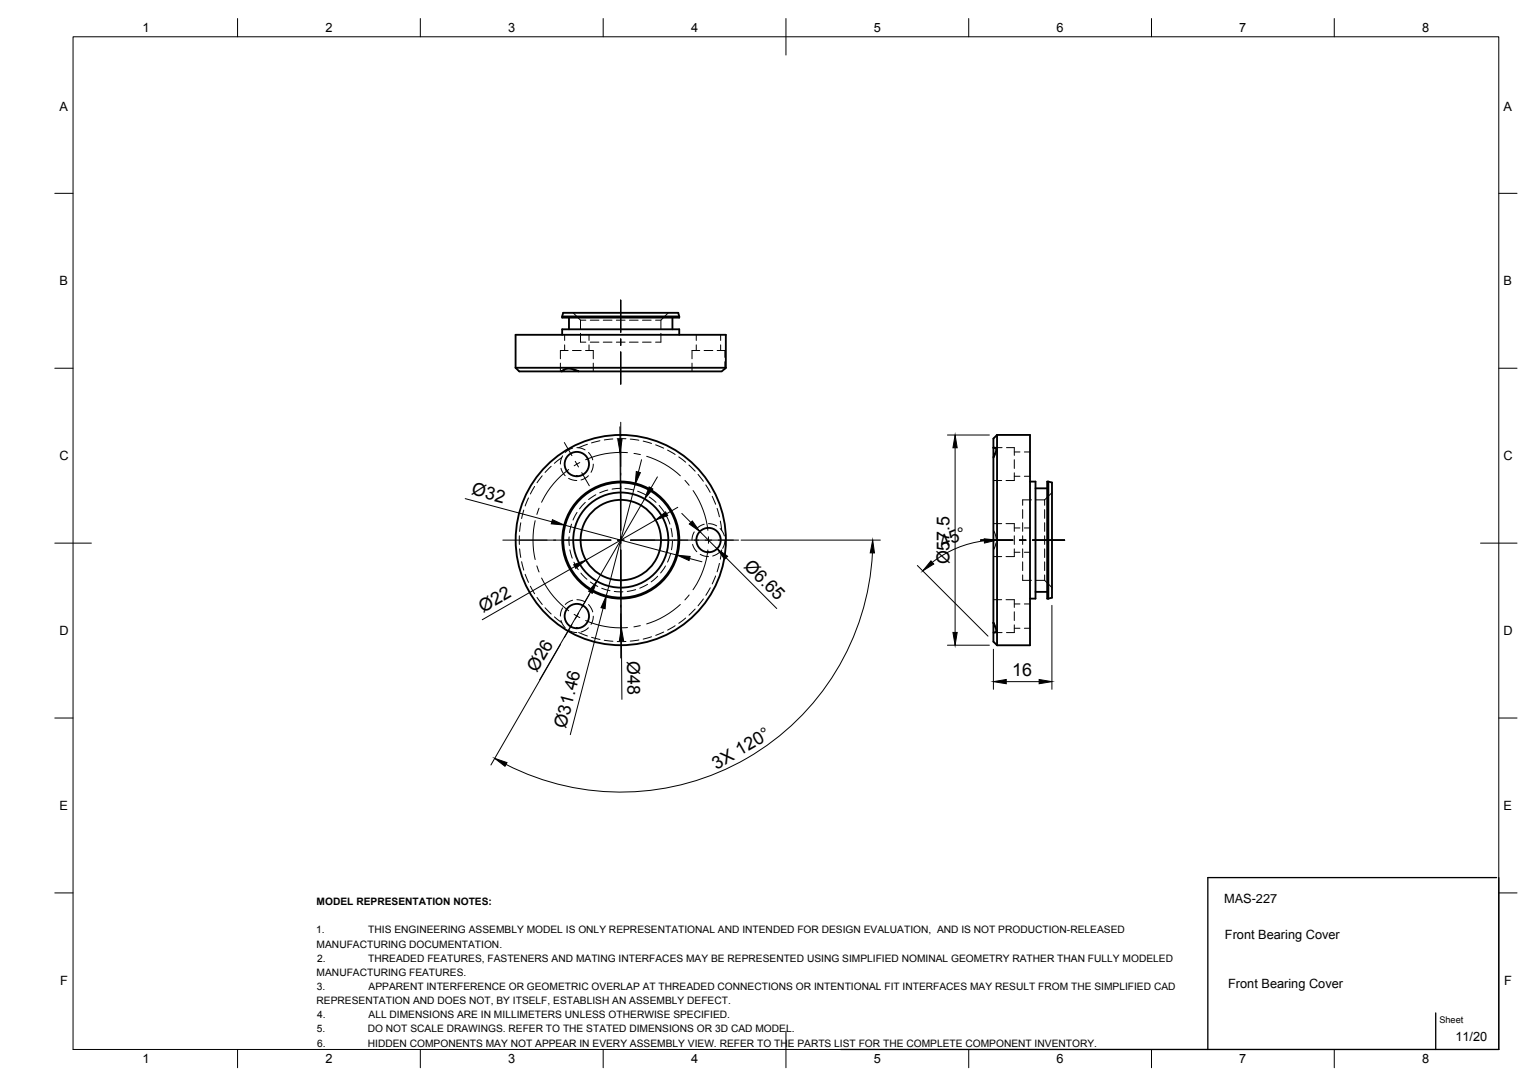
ISO-10303-21;
HEADER;
FILE_DESCRIPTION (('STEP AP214'),
    '1' );
FILE_NAME ( 'Front Bearing Cover.step', '2026-10-06T08:24:41', ( '' ), ( '' ), 'STEP AP214', 'Unspecified', '' );
FILE_SCHEMA (( 'AUTOMOTIVE_DESIGN' ));
ENDSEC;
DATA;
#2=LINE ( 'NONE', #16920, #12528 ) ;
#50=AXIS2_PLACEMENT_3D ( 'NONE', #26604, #25051, #22376 ) ;
#52=VECTOR ( 'NONE', #14977, 39.37007874015748143 ) ;
#127=DIRECTION ( 'NONE',  ( -1.000000000000000000, 0.000000000000000000, 0.000000000000000000 ) ) ;
#158=VERTEX_POINT ( 'NONE', #15724 ) ;
#172=CARTESIAN_POINT ( 'NONE',  ( -0.6029881478123397809, 1.118968434182175953, 0.03326447829408156476 ) ) ;
#190=CARTESIAN_POINT ( 'NONE',  ( -0.6299212598425196763, -0.4724409448818898127, -0.8182917201112815953 ) ) ;
#192=DIRECTION ( 'NONE',  ( -1.000000000000000000, 0.000000000000000000, 0.000000000000000000 ) ) ;
#253=DIRECTION ( 'NONE',  ( -1.000000000000000000, 0.000000000000000000, 0.000000000000000000 ) ) ;
#272=EDGE_CURVE ( 'NONE', #27250, #26868, #24521, .T. ) ;
#312=DIRECTION ( 'NONE',  ( 0.000000000000000000, 0.000000000000000000, 1.000000000000000000 ) ) ;
#392=ORIENTED_EDGE ( 'NONE', *, *, #12058, .F. ) ;
#416=EDGE_CURVE ( 'NONE', #7640, #15191, #10471, .T. ) ;
#433=DIRECTION ( 'NONE',  ( 1.000000000000000000, 0.000000000000000000, 0.000000000000000000 ) ) ;
#441=DIRECTION ( 'NONE',  ( 1.000000000000000000, 0.000000000000000000, 0.000000000000000000 ) ) ;
#479=CYLINDRICAL_SURFACE ( 'NONE', #571, 0.5570866141732283561 ) ;
#480=AXIS2_PLACEMENT_3D ( 'NONE', #1585, #2519, #13258 ) ;
#513=ORIENTED_EDGE ( 'NONE', *, *, #2642, .T. ) ;
#528=EDGE_LOOP ( 'NONE', ( #9986, #24877, #1531, #26427 ) ) ;
#562=FACE_OUTER_BOUND ( 'NONE', #19020, .T. ) ;
#571=AXIS2_PLACEMENT_3D ( 'NONE', #26308, #7804, #10047 ) ;
#585=EDGE_CURVE ( 'NONE', #20760, #20801, #19125, .T. ) ;
#624=CARTESIAN_POINT ( 'NONE',  ( -0.6020308615105518513, -0.5839868939189144514, 0.9562171551411200454 ) ) ;
#670=AXIS2_PLACEMENT_3D ( 'NONE', #15079, #14812, #19294 ) ;
#698=CIRCLE ( 'NONE', #4312, 0.5570866141732283561 ) ;
#725=ORIENTED_EDGE ( 'NONE', *, *, #8155, .T. ) ;
#767=EDGE_CURVE ( 'NONE', #19729, #5602, #7540, .T. ) ;
#774=LINE ( 'NONE', #17967, #26208 ) ;
#782=CYLINDRICAL_SURFACE ( 'NONE', #20278, 0.4330708661417322913 ) ;
#838=EDGE_CURVE ( 'NONE', #4142, #1699, #4370, .T. ) ;
#875=EDGE_CURVE ( 'NONE', #4894, #7494, #21145, .T. ) ;
#905=CARTESIAN_POINT ( 'NONE',  ( -0.1771653543307086520, 0.5935039370078740717, 0.000000000000000000 ) ) ;
#906=ORIENTED_EDGE ( 'NONE', *, *, #6294, .T. ) ;
#913=FACE_OUTER_BOUND ( 'NONE', #10036, .T. ) ;
#918=VECTOR ( 'NONE', #23051, 39.37007874015748143 ) ;
#928=EDGE_CURVE ( 'NONE', #158, #23473, #6082, .T. ) ;
#936=AXIS2_PLACEMENT_3D ( 'NONE', #3031, #24513, #15779 ) ;
#939=CARTESIAN_POINT ( 'NONE',  ( -0.6299212598425196763, 1.087444635826771533, -0.1051828227901515783 ) ) ;
#940=FACE_OUTER_BOUND ( 'NONE', #528, .T. ) ;
#951=VECTOR ( 'NONE', #3285, 39.37007874015748143 ) ;
#1039=DIRECTION ( 'NONE',  ( 0.000000000000000000, 0.000000000000000000, 1.000000000000000000 ) ) ;
#1046=DIRECTION ( 'NONE',  ( 0.000000000000000000, 0.000000000000000000, 1.000000000000000000 ) ) ;
#1048=AXIS2_PLACEMENT_3D ( 'NONE', #23857, #19612, #2759 ) ;
#1080=CONICAL_SURFACE ( 'NONE', #17752, 0.6246466694403326469, 0.2617993874999998694 ) ;
#1092=ORIENTED_EDGE ( 'NONE', *, *, #1886, .F. ) ;
#1098=( NAMED_UNIT ( * ) PLANE_ANGLE_UNIT ( ) SI_UNIT ( $, .RADIAN. ) ) ;
#1120=FACE_OUTER_BOUND ( 'NONE', #1478, .T. ) ;
#1124=AXIS2_PLACEMENT_3D ( 'NONE', #13348, #15489, #11366 ) ;
#1198=DIRECTION ( 'NONE',  ( -1.000000000000000000, 0.000000000000000000, 0.000000000000000000 ) ) ;
#1239=CARTESIAN_POINT ( 'NONE',  ( -0.1141732283464566844, 0.000000000000000000, 0.000000000000000000 ) ) ;
#1283=VECTOR ( 'NONE', #10032, 39.37007874015748143 ) ;
#1301=AXIS2_PLACEMENT_3D ( 'NONE', #19572, #253, #4583 ) ;
#1342=VERTEX_POINT ( 'NONE', #2206 ) ;
#1346=ORIENTED_EDGE ( 'NONE', *, *, #7162, .F. ) ;
#1382=DIRECTION ( 'NONE',  ( -1.000000000000000000, 0.000000000000000000, 0.000000000000000000 ) ) ;
#1478=EDGE_LOOP ( 'NONE', ( #8404, #19161 ) ) ;
#1485=ORIENTED_EDGE ( 'NONE', *, *, #4157, .T. ) ;
#1531=ORIENTED_EDGE ( 'NONE', *, *, #24469, .T. ) ;
#1570=DIRECTION ( 'NONE',  ( 1.000000000000000000, 0.000000000000000000, 0.000000000000000000 ) ) ;
#1571=CIRCLE ( 'NONE', #24136, 0.1771653543307086798 ) ;
#1585=CARTESIAN_POINT ( 'NONE',  ( -0.1771653543307086520, 0.000000000000000000, 0.000000000000000000 ) ) ;
#1644=FACE_OUTER_BOUND ( 'NONE', #10088, .T. ) ;
#1657=PRODUCT_CONTEXT ( 'NONE', #12864, 'mechanical' ) ;
#1699=VERTEX_POINT ( 'NONE', #13055 ) ;
#1701=DIRECTION ( 'NONE',  ( -0.9659258263664939337, -0.2588190448135644917, 0.000000000000000000 ) ) ;
#1711=ORIENTED_EDGE ( 'NONE', *, *, #11780, .F. ) ;
#1740=CARTESIAN_POINT ( 'NONE',  ( -0.6071192803969113205, -0.6030946203081917201, -0.9382345488190140248 ) ) ;
#1753=CIRCLE ( 'NONE', #25681, 0.5118110236220472231 ) ;
#1777=CARTESIAN_POINT ( 'NONE',  ( 2.632951206231566310, -0.4724409448818898127, 0.6874452634183660926 ) ) ;
#1827=FACE_OUTER_BOUND ( 'NONE', #23500, .T. ) ;
#1877=DIRECTION ( 'NONE',  ( 0.000000000000000000, 0.000000000000000000, 1.000000000000000000 ) ) ;
#1881=CARTESIAN_POINT ( 'NONE',  ( -0.6138531223217379429, -0.4891464190266830436, -0.9948699164928014316 ) ) ;
#1886=EDGE_CURVE ( 'NONE', #7494, #4592, #5665, .T. ) ;
#1902=CARTESIAN_POINT ( 'NONE',  ( -0.6086685665488132946, -0.5056997808540499850, 0.9923580223642571863 ) ) ;
#1968=CARTESIAN_POINT ( 'NONE',  ( -0.6299212598425196763, -0.4724409448818898127, 0.6411263657805708061 ) ) ;
#1969=DIRECTION ( 'NONE',  ( 0.000000000000000000, 1.000000000000000000, 0.000000000000000000 ) ) ;
#1976=ORIENTED_EDGE ( 'NONE', *, *, #15552, .T. ) ;
#1989=CARTESIAN_POINT ( 'NONE',  ( -0.6299212598425196763, -1.092519685074702762, 0.000000000000000000 ) ) ;
#1992=CYLINDRICAL_SURFACE ( 'NONE', #10340, 0.1771653543307086798 ) ;
#2006=CARTESIAN_POINT ( 'NONE',  ( -0.2066929133858267931, 0.6299212598425196763, 0.000000000000000000 ) ) ;
#2020=AXIS2_PLACEMENT_3D ( 'NONE', #5757, #7869, #12099 ) ;
#2023=CARTESIAN_POINT ( 'NONE',  ( -0.6205631318075456315, -0.4724394499398413827, -0.9954595798869798617 ) ) ;
#2029=DIMENSIONAL_EXPONENTS ( 1.000000000000000000, 0.000000000000000000, 0.000000000000000000, 0.000000000000000000, 0.000000000000000000, 0.000000000000000000, 0.000000000000000000 ) ;
#2047=ORIENTED_EDGE ( 'NONE', *, *, #11733, .T. ) ;
#2096=ORIENTED_EDGE ( 'NONE', *, *, #13801, .T. ) ;
#2101=CARTESIAN_POINT ( 'NONE',  ( -0.3149606299212598381, 0.000000000000000000, 0.000000000000000000 ) ) ;
#2149=EDGE_CURVE ( 'NONE', #23473, #158, #698, .T. ) ;
#2157=ORIENTED_EDGE ( 'NONE', *, *, #18019, .T. ) ;
#2175=EDGE_CURVE ( 'NONE', #3772, #3172, #5916, .T. ) ;
#2206=CARTESIAN_POINT ( 'NONE',  ( -0.6299212598425196763, -0.6348133144914134274, -0.8891632684400255782 ) ) ;
#2228=ORIENTED_EDGE ( 'NONE', *, *, #17985, .F. ) ;
#2241=CARTESIAN_POINT ( 'NONE',  ( -0.6003937007829848183, 1.122047244090071727, 1.315345636034250449E-15 ) ) ;
#2293=EDGE_CURVE ( 'NONE', #20801, #20760, #12897, .T. ) ;
#2306=LINE ( 'NONE', #17693, #23561 ) ;
#2317=VERTEX_POINT ( 'NONE', #19276 ) ;
#2319=CYLINDRICAL_SURFACE ( 'NONE', #1301, 0.1308464566929133932 ) ;
#2341=CYLINDRICAL_SURFACE ( 'NONE', #16764, 0.1308464566929133932 ) ;
#2355=FACE_OUTER_BOUND ( 'NONE', #2723, .T. ) ;
#2398=CARTESIAN_POINT ( 'NONE',  ( -0.5177165354330708347, -0.4724409448818898127, 0.6411263657805708061 ) ) ;
#2414=LINE ( 'NONE', #2006, #23718 ) ;
#2449=EDGE_CURVE ( 'NONE', #14962, #17328, #26863, .T. ) ;
#2473=ORIENTED_EDGE ( 'NONE', *, *, #20578, .F. ) ;
#2475=VECTOR ( 'NONE', #16821, 39.37007874015748143 ) ;
#2519=DIRECTION ( 'NONE',  ( 1.000000000000000000, 0.000000000000000000, 0.000000000000000000 ) ) ;
#2526=DIRECTION ( 'NONE',  ( 1.000000000000000000, 0.000000000000000000, 0.000000000000000000 ) ) ;
#2535=CARTESIAN_POINT ( 'NONE',  ( -0.6299212598425196763, -0.4526313213353582721, -0.9943460912301771426 ) ) ;
#2600=DIRECTION ( 'NONE',  ( 0.000000000000000000, 0.000000000000000000, 1.000000000000000000 ) ) ;
#2609=DIRECTION ( 'NONE',  ( 1.000000000000000000, 0.000000000000000000, 0.000000000000000000 ) ) ;
#2618=ORIENTED_EDGE ( 'NONE', *, *, #8797, .T. ) ;
#2630=CARTESIAN_POINT ( 'NONE',  ( -0.2362204724409449064, 0.9448818897637796255, 0.1308464566929133654 ) ) ;
#2635=ORIENTED_EDGE ( 'NONE', *, *, #16037, .F. ) ;
#2642=EDGE_CURVE ( 'NONE', #5602, #25182, #2, .T. ) ;
#2720=EDGE_CURVE ( 'NONE', #5602, #19729, #7100, .T. ) ;
#2723=EDGE_LOOP ( 'NONE', ( #26638, #22078, #16466, #23009 ) ) ;
#2759=DIRECTION ( 'NONE',  ( 0.000000000000000000, 0.000000000000000000, -1.000000000000000000 ) ) ;
#2778=EDGE_CURVE ( 'NONE', #26868, #27250, #21542, .T. ) ;
#2786=CARTESIAN_POINT ( 'NONE',  ( -0.03937007874015747977, 0.000000000000000000, 0.000000000000000000 ) ) ;
#2850=PLANE ( 'NONE',  #16081 ) ;
#2955=CYLINDRICAL_SURFACE ( 'NONE', #4382, 0.6299212598425196763 ) ;
#2956=ADVANCED_FACE ( 'NONE', ( #9507, #11506 ), #18107, .T. ) ;
#3017=ORIENTED_EDGE ( 'NONE', *, *, #6004, .T. ) ;
#3031=CARTESIAN_POINT ( 'NONE',  ( -0.05118110236220472370, 0.000000000000000000, 0.000000000000000000 ) ) ;
#3041=DIRECTION ( 'NONE',  ( 0.000000000000000000, 1.000000000000000000, 0.000000000000000000 ) ) ;
#3045=SURFACE_SIDE_STYLE ('',( #5177 ) ) ;
#3076=MANIFOLD_SOLID_BREP ( 'Front Bearing Cover', #11437 ) ;
#3092=DIRECTION ( 'NONE',  ( 0.000000000000000000, 1.000000000000000000, 0.000000000000000000 ) ) ;
#3147=FACE_OUTER_BOUND ( 'NONE', #4581, .T. ) ;
#3157=PRODUCT_DEFINITION_CONTEXT ( 'detailed design', #6031, 'design' ) ;
#3162=DIRECTION ( 'NONE',  ( 0.7071067818211385081, 0.7071067805519564153, -8.659560554583433905E-17 ) ) ;
#3165=AXIS2_PLACEMENT_3D ( 'NONE', #26491, #11954, #22410 ) ;
#3169=DIRECTION ( 'NONE',  ( 0.000000000000000000, 0.000000000000000000, 1.000000000000000000 ) ) ;
#3172=VERTEX_POINT ( 'NONE', #20257 ) ;
#3176=ORIENTED_EDGE ( 'NONE', *, *, #19126, .T. ) ;
#3186=CYLINDRICAL_SURFACE ( 'NONE', #8980, 0.5570866141732283561 ) ;
#3280=CIRCLE ( 'NONE', #22700, 0.1771653543307086798 ) ;
#3285=DIRECTION ( 'NONE',  ( -1.000000000000000000, 0.000000000000000000, 0.000000000000000000 ) ) ;
#3289=ORIENTED_EDGE ( 'NONE', *, *, #7803, .T. ) ;
#3334=CARTESIAN_POINT ( 'NONE',  ( 1.857656692913385893E-16, 0.6193720790381457286, 7.649715443242610847E-17 ) ) ;
#3339=AXIS2_PLACEMENT_3D ( 'NONE', #27556, #6091, #1969 ) ;
#3421=PLANE ( 'NONE',  #6401 ) ;
#3458=CARTESIAN_POINT ( 'NONE',  ( -0.07874015748031495954, 0.000000000000000000, 0.000000000000000000 ) ) ;
#3556=CARTESIAN_POINT ( 'NONE',  ( -0.02559055118110236185, -0.6299212598425196763, 7.714310545810098438E-17 ) ) ;
#3561=DIRECTION ( 'NONE',  ( -1.000000000000000000, 0.000000000000000000, 0.000000000000000000 ) ) ;
#3634=CARTESIAN_POINT ( 'NONE',  ( -0.5905511811023621549, 0.000000000000000000, 0.000000000000000000 ) ) ;
#3665=DIRECTION ( 'NONE',  ( 0.000000000000000000, 0.000000000000000000, 1.000000000000000000 ) ) ;
#3691=PRODUCT ( 'Front Bearing Cover', 'Front Bearing Cover', '', ( #1657 ) ) ;
#3700=VECTOR ( 'NONE', #23424, 39.37007874015748143 ) ;
#3772=VERTEX_POINT ( 'NONE', #20861 ) ;
#3862=CARTESIAN_POINT ( 'NONE',  ( -0.6086690512655491547, -0.5056979702033415069, -0.9923584033843172447 ) ) ;
#3879=EDGE_CURVE ( 'NONE', #13155, #23967, #1753, .T. ) ;
#3884=ORIENTED_EDGE ( 'NONE', *, *, #5984, .T. ) ;
#3919=CARTESIAN_POINT ( 'NONE',  ( -0.2362204724409449064, -1.131889763779527547, 1.386165176200252194E-16 ) ) ;
#3977=CARTESIAN_POINT ( 'NONE',  ( -0.4055118110236220486, -0.4724409448818898127, -0.8182917201112815953 ) ) ;
#4009=CARTESIAN_POINT ( 'NONE',  ( -0.6050289243185338339, -0.5969388012301621860, -0.9446411342989878834 ) ) ;
#4010=AXIS2_PLACEMENT_3D ( 'NONE', #17654, #27861, #13413 ) ;
#4032=EDGE_LOOP ( 'NONE', ( #13615, #17061 ) ) ;
#4033=ORIENTED_EDGE ( 'NONE', *, *, #2149, .F. ) ;
#4039=AXIS2_PLACEMENT_3D ( 'NONE', #2786, #15416, #312 ) ;
#4052=DIRECTION ( 'NONE',  ( 0.000000000000000000, -1.000000000000000000, 0.000000000000000000 ) ) ;
#4058=ORIENTED_EDGE ( 'NONE', *, *, #13801, .F. ) ;
#4088=CARTESIAN_POINT ( 'NONE',  ( -0.05118110236220472370, 0.5570866141732283561, 0.000000000000000000 ) ) ;
#4100=AXIS2_PLACEMENT_3D ( 'NONE', #11265, #13943, #7163 ) ;
#4142=VERTEX_POINT ( 'NONE', #15662 ) ;
#4157=EDGE_CURVE ( 'NONE', #15892, #26494, #5820, .T. ) ;
#4227=DIRECTION ( 'NONE',  ( 1.000000000000000000, 0.000000000000000000, 0.000000000000000000 ) ) ;
#4284=ORIENTED_EDGE ( 'NONE', *, *, #8725, .T. ) ;
#4304=DIRECTION ( 'NONE',  ( -1.000000000000000000, 0.000000000000000000, 0.000000000000000000 ) ) ;
#4311=EDGE_CURVE ( 'NONE', #19874, #10834, #13049, .T. ) ;
#4312=AXIS2_PLACEMENT_3D ( 'NONE', #13964, #10269, #16225 ) ;
#4370=LINE ( 'NONE', #13117, #25467 ) ;
#4382=AXIS2_PLACEMENT_3D ( 'NONE', #11586, #24576, #3092 ) ;
#4397=ADVANCED_FACE ( 'NONE', ( #21355 ), #1992, .F. ) ;
#4430=CARTESIAN_POINT ( 'NONE',  ( -0.6299212598425196763, 1.087444635826771533, -0.1051828227901515783 ) ) ;
#4453=ORIENTED_EDGE ( 'NONE', *, *, #16423, .F. ) ;
#4499=CARTESIAN_POINT ( 'NONE',  ( -0.6299212598425196763, 0.000000000000000000, 0.000000000000000000 ) ) ;
#4523=CARTESIAN_POINT ( 'NONE',  ( -0.6299212598425196763, 0.000000000000000000, 0.000000000000000000 ) ) ;
#4564=DIRECTION ( 'NONE',  ( -1.000000000000000000, 0.000000000000000000, 0.000000000000000000 ) ) ;
#4581=EDGE_LOOP ( 'NONE', ( #20664, #22877 ) ) ;
#4583=DIRECTION ( 'NONE',  ( 0.000000000000000000, 0.000000000000000000, -1.000000000000000000 ) ) ;
#4592=VERTEX_POINT ( 'NONE', #13879 ) ;
#4629=AXIS2_PLACEMENT_3D ( 'NONE', #11749, #5251, #25164 ) ;
#4647=ORIENTED_EDGE ( 'NONE', *, *, #24298, .T. ) ;
#4661=DIRECTION ( 'NONE',  ( -1.000000000000000000, 0.000000000000000000, 0.000000000000000000 ) ) ;
#4671=CIRCLE ( 'NONE', #19590, 1.131889763779527547 ) ;
#4677=CYLINDRICAL_SURFACE ( 'NONE', #19084, 0.1308464566929133932 ) ;
#4704=ORIENTED_EDGE ( 'NONE', *, *, #272, .F. ) ;
#4711=FACE_OUTER_BOUND ( 'NONE', #27003, .T. ) ;
#4795=VERTEX_POINT ( 'NONE', #8631 ) ;
#4815=ORIENTED_EDGE ( 'NONE', *, *, #20578, .T. ) ;
#4843=CARTESIAN_POINT ( 'NONE',  ( -0.6002206662457667541, -0.5625442442678819654, 0.9710808210061889767 ) ) ;
#4867=MECHANICAL_DESIGN_GEOMETRIC_PRESENTATION_REPRESENTATION('',(#9349),#13888);
#4879=EDGE_LOOP ( 'NONE', ( #13228, #15107, #14974, #9118 ) ) ;
#4894=VERTEX_POINT ( 'NONE', #6696 ) ;
#4897=CIRCLE ( 'NONE', #4010, 0.1308464566929133932 ) ;
#4929=AXIS2_PLACEMENT_3D ( 'NONE', #19766, #433, #15543 ) ;
#4945=DIRECTION ( 'NONE',  ( -1.000000000000000000, 0.000000000000000000, 0.000000000000000000 ) ) ;
#5070=CARTESIAN_POINT ( 'NONE',  ( -0.2362204724409449064, 1.131889763779527547, 0.000000000000000000 ) ) ;
#5085=AXIS2_PLACEMENT_3D ( 'NONE', #24163, #22043, #26013 ) ;
#5128=DIRECTION ( 'NONE',  ( 0.000000000000000000, 0.000000000000000000, -1.000000000000000000 ) ) ;
#5156=CARTESIAN_POINT ( 'NONE',  ( -0.6209926255554318875, 1.097802432539390916, -0.08994119036278866441 ) ) ;
#5177=SURFACE_STYLE_FILL_AREA ( #25489 ) ;
#5196=DIRECTION ( 'NONE',  ( 0.000000000000000000, -1.000000000000000000, 0.000000000000000000 ) ) ;
#5229=CARTESIAN_POINT ( 'NONE',  ( 0.000000000000000000, 0.000000000000000000, 0.000000000000000000 ) ) ;
#5246=ORIENTED_EDGE ( 'NONE', *, *, #416, .F. ) ;
#5251=DIRECTION ( 'NONE',  ( -1.000000000000000000, 0.000000000000000000, 0.000000000000000000 ) ) ;
#5303=CARTESIAN_POINT ( 'NONE',  ( -0.6130487771524342211, 1.107101695598143642, -0.07148403028289961048 ) ) ;
#5379=DIRECTION ( 'NONE',  ( -1.000000000000000000, 0.000000000000000000, 0.000000000000000000 ) ) ;
#5451=ORIENTED_EDGE ( 'NONE', *, *, #16037, .T. ) ;
#5452=EDGE_LOOP ( 'NONE', ( #15442, #19741 ) ) ;
#5489=VERTEX_POINT ( 'NONE', #18159 ) ;
#5490=CARTESIAN_POINT ( 'NONE',  ( 1.877524803149606209E-16, 5.303588500244442984E-17, -0.4330708661417322913 ) ) ;
#5519=ORIENTED_EDGE ( 'NONE', *, *, #12634, .F. ) ;
#5566=CARTESIAN_POINT ( 'NONE',  ( -0.02559055118110236185, 0.000000000000000000, 0.000000000000000000 ) ) ;
#5575=CARTESIAN_POINT ( 'NONE',  ( -0.07874015748031495954, 0.000000000000000000, 0.4330708661417322913 ) ) ;
#5596=DIRECTION ( 'NONE',  ( -1.000000000000000000, 0.000000000000000000, 0.000000000000000000 ) ) ;
#5602=VERTEX_POINT ( 'NONE', #3334 ) ;
#5617=EDGE_CURVE ( 'NONE', #9929, #1699, #22039, .T. ) ;
#5633=FACE_BOUND ( 'NONE', #5452, .T. ) ;
#5639=VECTOR ( 'NONE', #127, 39.37007874015748143 ) ;
#5665=CIRCLE ( 'NONE', #24152, 0.1771653543307086520 ) ;
#5671=ORIENTED_EDGE ( 'NONE', *, *, #9315, .F. ) ;
#5727=ORIENTED_EDGE ( 'NONE', *, *, #19126, .F. ) ;
#5757=CARTESIAN_POINT ( 'NONE',  ( -0.6299212598425196763, 0.9448818897637796255, -9.561468503937007847E-18 ) ) ;
#5784=VERTEX_POINT ( 'NONE', #18914 ) ;
#5798=DIRECTION ( 'NONE',  ( 0.7071067818211390632, -8.659560554583428975E-17, -0.7071067805519560823 ) ) ;
#5817=AXIS2_PLACEMENT_3D ( 'NONE', #2101, #10713, #12965 ) ;
#5820=CIRCLE ( 'NONE', #13027, 0.6299212598425196763 ) ;
#5827=VERTEX_POINT ( 'NONE', #1968 ) ;
#5856=LINE ( 'NONE', #7831, #22622 ) ;
#5895=FACE_BOUND ( 'NONE', #4032, .T. ) ;
#5916=LINE ( 'NONE', #5490, #20087 ) ;
#5984=EDGE_CURVE ( 'NONE', #10834, #19874, #22524, .T. ) ;
#6004=EDGE_CURVE ( 'NONE', #27250, #20760, #8800, .T. ) ;
#6031=APPLICATION_CONTEXT ( 'automotive_design' ) ;
#6082=CIRCLE ( 'NONE', #3339, 0.5570866141732283561 ) ;
#6091=DIRECTION ( 'NONE',  ( 1.000000000000000000, 0.000000000000000000, 0.000000000000000000 ) ) ;
#6114=EDGE_LOOP ( 'NONE', ( #20873, #27817 ) ) ;
#6130=CIRCLE ( 'NONE', #15600, 0.6299212598425196763 ) ;
#6134=CIRCLE ( 'NONE', #20997, 0.6299212598425196763 ) ;
#6141=CARTESIAN_POINT ( 'NONE',  ( -0.6010693932361863556, -0.5770964849832589394, -0.9615141454542482924 ) ) ;
#6152=ORIENTED_EDGE ( 'NONE', *, *, #19042, .F. ) ;
#6181=B_SPLINE_CURVE_WITH_KNOTS ( 'NONE', 3,
 ( #10656, #23399, #12643, #21270, #1902, #19277, #10515, #19134, #27768, #4843, #19830, #624, #17697, #13186, #17432, #26050, #15347 ),
 .UNSPECIFIED., .F., .F.,
 ( 4, 2, 2, 1, 2, 2, 2, 2, 4 ),
 ( 0.08984410251848014284, 0.2036135897036702169, 0.2604983332962649833, 0.3173830768888596943, 0.4311525640740497822, 0.5449220512592398702, 0.6586915384444299582, 0.7724610256296200461, 1.000000000000000000 ),
 .UNSPECIFIED. ) ;
#6196=FACE_OUTER_BOUND ( 'NONE', #21586, .T. ) ;
#6214=EDGE_CURVE ( 'NONE', #25955, #13695, #25285, .T. ) ;
#6222=CARTESIAN_POINT ( 'NONE',  ( -0.6042043723480865491, 1.117528104686773327, 0.04027680511324581436 ) ) ;
#6269=DIRECTION ( 'NONE',  ( 1.000000000000000000, 0.000000000000000000, 0.000000000000000000 ) ) ;
#6281=ADVANCED_FACE ( 'NONE', ( #12240 ), #3186, .T. ) ;
#6294=EDGE_CURVE ( 'NONE', #5784, #2317, #11684, .T. ) ;
#6306=DIRECTION ( 'NONE',  ( 0.000000000000000000, 0.000000000000000000, 1.000000000000000000 ) ) ;
#6348=CARTESIAN_POINT ( 'NONE',  ( 2.632951206231566310, 0.9448818897637796255, -0.1308464566929134210 ) ) ;
#6370=ORIENTED_EDGE ( 'NONE', *, *, #25909, .F. ) ;
#6401=AXIS2_PLACEMENT_3D ( 'NONE', #11778, #20397, #18398 ) ;
#6426=DIRECTION ( 'NONE',  ( -1.000000000000000000, 0.000000000000000000, 0.000000000000000000 ) ) ;
#6443=DIRECTION ( 'NONE',  ( 0.000000000000000000, 0.000000000000000000, -1.000000000000000000 ) ) ;
#6452=DIRECTION ( 'NONE',  ( -0.9659258263664939337, 0.2588190448135644917, 3.169619147893071122E-17 ) ) ;
#6487=ADVANCED_FACE ( 'NONE', ( #7002 ), #8554, .T. ) ;
#6551=DIRECTION ( 'NONE',  ( -1.000000000000000000, 0.000000000000000000, 0.000000000000000000 ) ) ;
#6575=ADVANCED_FACE ( 'NONE', ( #11096 ), #782, .F. ) ;
#6696=CARTESIAN_POINT ( 'NONE',  ( -0.6003937007829848183, 1.122047244090071727, 1.315345636034250449E-15 ) ) ;
#6708=DIRECTION ( 'NONE',  ( 1.000000000000000000, 0.000000000000000000, 0.000000000000000000 ) ) ;
#6710=CARTESIAN_POINT ( 'NONE',  ( -0.4055118110236220486, -0.4724409448818898127, 0.8182917201112794858 ) ) ;
#6771=ORIENTED_EDGE ( 'NONE', *, *, #12058, .T. ) ;
#6778=DIRECTION ( 'NONE',  ( 0.000000000000000000, 1.000000000000000000, 0.000000000000000000 ) ) ;
#6781=FACE_OUTER_BOUND ( 'NONE', #9892, .T. ) ;
#6790=ORIENTED_EDGE ( 'NONE', *, *, #21213, .T. ) ;
#6805=EDGE_CURVE ( 'NONE', #12305, #4795, #15787, .T. ) ;
#6813=ORIENTED_EDGE ( 'NONE', *, *, #4157, .F. ) ;
#6821=ORIENTED_EDGE ( 'NONE', *, *, #10361, .T. ) ;
#6866=ORIENTED_EDGE ( 'NONE', *, *, #9739, .T. ) ;
#6895=LINE ( 'NONE', #15525, #20299 ) ;
#6932=CIRCLE ( 'NONE', #7357, 0.5570866141732283561 ) ;
#6950=VECTOR ( 'NONE', #5798, 39.37007874015748143 ) ;
#6998=DIRECTION ( 'NONE',  ( 0.000000000000000000, 0.000000000000000000, -1.000000000000000000 ) ) ;
#7002=FACE_OUTER_BOUND ( 'NONE', #15517, .T. ) ;
#7024=CARTESIAN_POINT ( 'NONE',  ( -0.2066929133858267931, 0.000000000000000000, 0.000000000000000000 ) ) ;
#7061=ORIENTED_EDGE ( 'NONE', *, *, #8900, .T. ) ;
#7074=CARTESIAN_POINT ( 'NONE',  ( -0.5905511811023621549, -1.131889763779527547, 1.386165176200252194E-16 ) ) ;
#7082=EDGE_CURVE ( 'NONE', #4795, #4592, #6895, .T. ) ;
#7100=CIRCLE ( 'NONE', #14817, 0.6193720790381457286 ) ;
#7102=DIRECTION ( 'NONE',  ( -1.000000000000000000, 0.000000000000000000, 0.000000000000000000 ) ) ;
#7143=CARTESIAN_POINT ( 'NONE',  ( -0.6205616028481958368, -0.4724399524669597450, 0.9954595399567032210 ) ) ;
#7152=AXIS2_PLACEMENT_3D ( 'NONE', #15250, #21737, #17080 ) ;
#7162=EDGE_CURVE ( 'NONE', #26868, #20801, #19748, .T. ) ;
#7163=DIRECTION ( 'NONE',  ( 0.000000000000000000, 0.000000000000000000, 1.000000000000000000 ) ) ;
#7234=ADVANCED_FACE ( 'NONE', ( #13652 ), #26641, .F. ) ;
#7238=CARTESIAN_POINT ( 'NONE',  ( -0.4055118110236220486, -0.4724409448818898127, -0.6411263657805729155 ) ) ;
#7241=DIRECTION ( 'NONE',  ( 0.000000000000000000, 0.000000000000000000, 1.000000000000000000 ) ) ;
#7288=FACE_OUTER_BOUND ( 'NONE', #19185, .T. ) ;
#7315=ORIENTED_EDGE ( 'NONE', *, *, #2449, .F. ) ;
#7339=ADVANCED_FACE ( 'NONE', ( #23454 ), #23862, .T. ) ;
#7344=UNCERTAINTY_MEASURE_WITH_UNIT (LENGTH_MEASURE( 1.000000000000000082E-05 ), #9669, 'distance_accuracy_value', 'NONE') ;
#7357=AXIS2_PLACEMENT_3D ( 'NONE', #26685, #22598, #20624 ) ;
#7370=AXIS2_PLACEMENT_3D ( 'NONE', #26123, #20035, #6778 ) ;
#7395=DIRECTION ( 'NONE',  ( 0.000000000000000000, 1.000000000000000000, 0.000000000000000000 ) ) ;
#7418=CARTESIAN_POINT ( 'NONE',  ( -0.6094642026423211512, 1.111319899719084070, -0.06074667524627151011 ) ) ;
#7467=EDGE_LOOP ( 'NONE', ( #24320, #21051, #7570, #16923 ) ) ;
#7470=AXIS2_PLACEMENT_3D ( 'NONE', #26049, #6708, #21959 ) ;
#7494=VERTEX_POINT ( 'NONE', #12093 ) ;
#7510=CARTESIAN_POINT ( 'NONE',  ( 2.632951206231566310, -0.4724409448818898127, 0.9491381768041928790 ) ) ;
#7515=FACE_OUTER_BOUND ( 'NONE', #21445, .T. ) ;
#7540=CIRCLE ( 'NONE', #17030, 0.6193720790381457286 ) ;
#7541=CARTESIAN_POINT ( 'NONE',  ( -0.07874015748031495954, 0.000000000000000000, 0.000000000000000000 ) ) ;
#7566=ORIENTED_EDGE ( 'NONE', *, *, #15556, .F. ) ;
#7570=ORIENTED_EDGE ( 'NONE', *, *, #18019, .F. ) ;
#7610=SHAPE_REPRESENTATION_RELATIONSHIP ( 'NONE' , 'NONE' ,  #24703, #14395 ) ;
#7612=DIRECTION ( 'NONE',  ( -1.000000000000000000, 0.000000000000000000, 0.000000000000000000 ) ) ;
#7613=FACE_BOUND ( 'NONE', #22127, .T. ) ;
#7618=AXIS2_PLACEMENT_3D ( 'NONE', #20287, #5596, #13787 ) ;
#7623=DIRECTION ( 'NONE',  ( 0.000000000000000000, 0.000000000000000000, 1.000000000000000000 ) ) ;
#7640=VERTEX_POINT ( 'NONE', #10111 ) ;
#7646=ORIENTED_EDGE ( 'NONE', *, *, #15688, .T. ) ;
#7659=ORIENTED_EDGE ( 'NONE', *, *, #17985, .T. ) ;
#7686=ORIENTED_EDGE ( 'NONE', *, *, #1886, .T. ) ;
#7730=FACE_OUTER_BOUND ( 'NONE', #4879, .T. ) ;
#7758=ORIENTED_EDGE ( 'NONE', *, *, #8296, .F. ) ;
#7761=ORIENTED_EDGE ( 'NONE', *, *, #3879, .T. ) ;
#7781=ORIENTED_EDGE ( 'NONE', *, *, #16423, .T. ) ;
#7803=EDGE_CURVE ( 'NONE', #23473, #5489, #774, .T. ) ;
#7804=DIRECTION ( 'NONE',  ( 1.000000000000000000, 0.000000000000000000, 0.000000000000000000 ) ) ;
#7831=CARTESIAN_POINT ( 'NONE',  ( -0.5177165354330708347, -0.4724409448818898127, 0.9954570744419881656 ) ) ;
#7835=ORIENTED_EDGE ( 'NONE', *, *, #23596, .F. ) ;
#7869=DIRECTION ( 'NONE',  ( 1.000000000000000000, 0.000000000000000000, 0.000000000000000000 ) ) ;
#7920=ORIENTED_EDGE ( 'NONE', *, *, #18017, .F. ) ;
#7923=DIRECTION ( 'NONE',  ( 1.000000000000000000, 0.000000000000000000, 0.000000000000000000 ) ) ;
#7971=CARTESIAN_POINT ( 'NONE',  ( 1.877524803149606209E-16, 0.000000000000000000, 0.4330708661417322913 ) ) ;
#7983=EDGE_CURVE ( 'NONE', #9494, #9714, #22658, .T. ) ;
#8014=CYLINDRICAL_SURFACE ( 'NONE', #670, 0.1308464566929133932 ) ;
#8030=DIRECTION ( 'NONE',  ( 0.000000000000000000, 0.000000000000000000, -1.000000000000000000 ) ) ;
#8056=ADVANCED_FACE ( 'NONE', ( #22520, #3147 ), #3421, .T. ) ;
#8095=ORIENTED_EDGE ( 'NONE', *, *, #19515, .T. ) ;
#8148=CARTESIAN_POINT ( 'NONE',  ( -0.4055118110236220486, 0.9448818897637796255, -9.561468503937007847E-18 ) ) ;
#8155=EDGE_CURVE ( 'NONE', #15191, #14962, #24958, .T. ) ;
#8198=CARTESIAN_POINT ( 'NONE',  ( -0.6205631318075456315, -0.4724394499398413827, -0.9954595798869798617 ) ) ;
#8269=ORIENTED_EDGE ( 'NONE', *, *, #875, .T. ) ;
#8296=EDGE_CURVE ( 'NONE', #9494, #3772, #13594, .T. ) ;
#8304=EDGE_LOOP ( 'NONE', ( #11579, #14620 ) ) ;
#8357=EDGE_LOOP ( 'NONE', ( #13425, #7835 ) ) ;
#8364=VERTEX_POINT ( 'NONE', #20677 ) ;
#8384=CARTESIAN_POINT ( 'NONE',  ( 1.857656692913385893E-16, 0.000000000000000000, 0.000000000000000000 ) ) ;
#8390=CARTESIAN_POINT ( 'NONE',  ( -0.6169742724477221829, -0.4807970751196540271, -0.9954635886630591735 ) ) ;
#8404=ORIENTED_EDGE ( 'NONE', *, *, #13633, .T. ) ;
#8421=EDGE_CURVE ( 'NONE', #19774, #15164, #5856, .T. ) ;
#8448=CARTESIAN_POINT ( 'NONE',  ( -0.4330708661417322913, -1.131889763779527547, 1.386165176200252194E-16 ) ) ;
#8451=EDGE_LOOP ( 'NONE', ( #8095, #26361, #25830, #21519, #13372, #6790, #725, #15217 ) ) ;
#8454=DIRECTION ( 'NONE',  ( 1.000000000000000000, 0.000000000000000000, 0.000000000000000000 ) ) ;
#8482=VERTEX_POINT ( 'NONE', #19112 ) ;
#8504=ORIENTED_EDGE ( 'NONE', *, *, #10361, .F. ) ;
#8538=ORIENTED_EDGE ( 'NONE', *, *, #18680, .T. ) ;
#8551=ORIENTED_EDGE ( 'NONE', *, *, #15454, .T. ) ;
#8554=CONICAL_SURFACE ( 'NONE', #27520, 0.6246466694403326469, 0.2617993874999998694 ) ;
#8631=CARTESIAN_POINT ( 'NONE',  ( -0.4055118110236220486, 0.9448818897637796255, 0.1771653543307086520 ) ) ;
#8652=ORIENTED_EDGE ( 'NONE', *, *, #9739, .F. ) ;
#8725=EDGE_CURVE ( 'NONE', #11982, #7640, #12720, .T. ) ;
#8797=EDGE_CURVE ( 'NONE', #15630, #25955, #27615, .T. ) ;
#8800=LINE ( 'NONE', #26305, #23461 ) ;
#8832=PLANE ( 'NONE',  #1124 ) ;
#8876=EDGE_LOOP ( 'NONE', ( #2228, #23043, #11268, #23391, #4453 ) ) ;
#8900=EDGE_CURVE ( 'NONE', #24768, #5827, #12722, .T. ) ;
#8905=ORIENTED_EDGE ( 'NONE', *, *, #23315, .T. ) ;
#8932=CARTESIAN_POINT ( 'NONE',  ( -0.6299212598425196763, 0.5659448818897637734, 0.000000000000000000 ) ) ;
#8980=AXIS2_PLACEMENT_3D ( 'NONE', #1239, #25235, #11676 ) ;
#9033=CARTESIAN_POINT ( 'NONE',  ( -0.6299212598425196763, 0.9448818897637796255, -0.1771653543307086520 ) ) ;
#9053=CARTESIAN_POINT ( 'NONE',  ( -0.4055118110236220486, -0.4724409448818898127, 0.6874452634183660926 ) ) ;
#9055=DIRECTION ( 'NONE',  ( -1.000000000000000000, 0.000000000000000000, 0.000000000000000000 ) ) ;
#9118=ORIENTED_EDGE ( 'NONE', *, *, #27438, .F. ) ;
#9122=CYLINDRICAL_SURFACE ( 'NONE', #1048, 0.1308464566929133932 ) ;
#9178=ORIENTED_EDGE ( 'NONE', *, *, #2293, .F. ) ;
#9185=VECTOR ( 'NONE', #23365, 39.37007874015748143 ) ;
#9232=AXIS2_PLACEMENT_3D ( 'NONE', #14485, #21352, #16444 ) ;
#9298=AXIS2_PLACEMENT_3D ( 'NONE', #4523, #2526, #17375 ) ;
#9315=EDGE_CURVE ( 'NONE', #17373, #26561, #25853, .T. ) ;
#9334=DIRECTION ( 'NONE',  ( -1.000000000000000000, 0.000000000000000000, 0.000000000000000000 ) ) ;
#9342=FACE_OUTER_BOUND ( 'NONE', #17613, .T. ) ;
#9349=STYLED_ITEM ( 'NONE', ( #13806 ), #3076 ) ;
#9369=DIRECTION ( 'NONE',  ( -1.000000000000000000, 0.000000000000000000, 0.000000000000000000 ) ) ;
#9377=LINE ( 'NONE', #22536, #20792 ) ;
#9419=LENGTH_MEASURE_WITH_UNIT ( LENGTH_MEASURE( 0.02539999999999999897 ), #11839 ) ;
#9494=VERTEX_POINT ( 'NONE', #5575 ) ;
#9507=FACE_BOUND ( 'NONE', #14650, .T. ) ;
#9544=ADVANCED_FACE ( 'NONE', ( #14487 ), #23138, .T. ) ;
#9669=( CONVERSION_BASED_UNIT ( 'INCH', #9948 ) LENGTH_UNIT ( ) NAMED_UNIT ( #2029 ) ) ;
#9683=EDGE_CURVE ( 'NONE', #8364, #4142, #13196, .T. ) ;
#9714=VERTEX_POINT ( 'NONE', #18826 ) ;
#9724=ADVANCED_FACE ( 'NONE', ( #23659 ), #13314, .T. ) ;
#9739=EDGE_CURVE ( 'NONE', #25182, #25584, #14606, .T. ) ;
#9779=CIRCLE ( 'NONE', #26443, 0.1308464566929133932 ) ;
#9796=LINE ( 'NONE', #20539, #24199 ) ;
#9811=ORIENTED_EDGE ( 'NONE', *, *, #12663, .T. ) ;
#9816=CARTESIAN_POINT ( 'NONE',  ( -0.6265111856126519552, -0.4592309206878726902, 0.9950886776261921307 ) ) ;
#9854=AXIS2_PLACEMENT_3D ( 'NONE', #20591, #18448, #8030 ) ;
#9891=CIRCLE ( 'NONE', #10806, 1.131889763779527547 ) ;
#9892=EDGE_LOOP ( 'NONE', ( #11009, #2047, #13091, #7761 ) ) ;
#9904=CARTESIAN_POINT ( 'NONE',  ( -0.6299212598425196763, 0.000000000000000000, 0.000000000000000000 ) ) ;
#9915=DIRECTION ( 'NONE',  ( -1.000000000000000000, 0.000000000000000000, 0.000000000000000000 ) ) ;
#9929=VERTEX_POINT ( 'NONE', #20082 ) ;
#9948=LENGTH_MEASURE_WITH_UNIT ( LENGTH_MEASURE( 0.02539999999999999897 ), #16321 ) ;
#9966=ORIENTED_EDGE ( 'NONE', *, *, #5617, .T. ) ;
#9986=ORIENTED_EDGE ( 'NONE', *, *, #8296, .T. ) ;
#10022=DIRECTION ( 'NONE',  ( -1.000000000000000000, 0.000000000000000000, 0.000000000000000000 ) ) ;
#10032=DIRECTION ( 'NONE',  ( 1.000000000000000000, 0.000000000000000000, 0.000000000000000000 ) ) ;
#10036=EDGE_LOOP ( 'NONE', ( #11650, #17799, #17741, #12878 ) ) ;
#10047=DIRECTION ( 'NONE',  ( 0.000000000000000000, 1.000000000000000000, 0.000000000000000000 ) ) ;
#10081=CIRCLE ( 'NONE', #26770, 0.6299212598425196763 ) ;
#10084=ORIENTED_EDGE ( 'NONE', *, *, #19042, .T. ) ;
#10088=EDGE_LOOP ( 'NONE', ( #8504, #14497, #26757, #12288 ) ) ;
#10094=ORIENTED_EDGE ( 'NONE', *, *, #25062, .F. ) ;
#10099=CIRCLE ( 'NONE', #17327, 0.1771653543307086520 ) ;
#10111=CARTESIAN_POINT ( 'NONE',  ( -0.4055118110236220486, -0.4724409448818898127, -0.9954570744419902750 ) ) ;
#10138=ORIENTED_EDGE ( 'NONE', *, *, #13111, .F. ) ;
#10196=DIRECTION ( 'NONE',  ( 0.000000000000000000, 0.000000000000000000, 1.000000000000000000 ) ) ;
#10202=CARTESIAN_POINT ( 'NONE',  ( -0.6003336567877981533, -0.5548708040260077468, -0.9753554781213541469 ) ) ;
#10208=EDGE_CURVE ( 'NONE', #24768, #19774, #3280, .T. ) ;
#10211=DIRECTION ( 'NONE',  ( -1.000000000000000000, 0.000000000000000000, 0.000000000000000000 ) ) ;
#10253=( GEOMETRIC_REPRESENTATION_CONTEXT ( 3 ) GLOBAL_UNCERTAINTY_ASSIGNED_CONTEXT ( ( #26832 ) ) GLOBAL_UNIT_ASSIGNED_CONTEXT ( ( #24681, #20168, #18602 ) ) REPRESENTATION_CONTEXT ( 'NONE', 'WORKASPACE' ) ) ;
#10269=DIRECTION ( 'NONE',  ( 1.000000000000000000, 0.000000000000000000, 0.000000000000000000 ) ) ;
#10282=ORIENTED_EDGE ( 'NONE', *, *, #928, .F. ) ;
#10340=AXIS2_PLACEMENT_3D ( 'NONE', #19656, #4661, #19506 ) ;
#10351=CARTESIAN_POINT ( 'NONE',  ( -0.6098677386912745302, -0.5016113632408703005, -0.9930866184834644672 ) ) ;
#10361=EDGE_CURVE ( 'NONE', #4142, #8364, #25358, .T. ) ;
#10436=CARTESIAN_POINT ( 'NONE',  ( -0.01968503937007873988, 0.000000000000000000, 0.000000000000000000 ) ) ;
#10471=LINE ( 'NONE', #27868, #9185 ) ;
#10485=LINE ( 'NONE', #3556, #21909 ) ;
#10515=CARTESIAN_POINT ( 'NONE',  ( -0.6034159556099095711, -0.5269038574519832041, 0.9872771499260571959 ) ) ;
#10595=ORIENTED_EDGE ( 'NONE', *, *, #22601, .T. ) ;
#10628=CARTESIAN_POINT ( 'NONE',  ( -0.6205631318075456315, -0.4724394499398413827, -0.9954595798869798617 ) ) ;
#10648=ORIENTED_EDGE ( 'NONE', *, *, #8421, .F. ) ;
#10656=CARTESIAN_POINT ( 'NONE',  ( -0.6205616028481958368, -0.4724399524669597450, 0.9954595399567032210 ) ) ;
#10658=FACE_BOUND ( 'NONE', #16051, .T. ) ;
#10666=AXIS2_PLACEMENT_3D ( 'NONE', #24477, #13612, #5128 ) ;
#10668=DIRECTION ( 'NONE',  ( -1.000000000000000000, 0.000000000000000000, 0.000000000000000000 ) ) ;
#10695=VERTEX_POINT ( 'NONE', #15902 ) ;
#10710=ADVANCED_FACE ( 'NONE', ( #940 ), #11885, .F. ) ;
#10713=DIRECTION ( 'NONE',  ( 1.000000000000000000, 0.000000000000000000, 0.000000000000000000 ) ) ;
#10730=CARTESIAN_POINT ( 'NONE',  ( -0.6131838103401908713, 1.106933345738153607, 0.07395176699543236365 ) ) ;
#10747=CARTESIAN_POINT ( 'NONE',  ( -0.2362204724409449064, -0.6299212598425196763, 7.714310545810098438E-17 ) ) ;
#10806=AXIS2_PLACEMENT_3D ( 'NONE', #3634, #24973, #5196 ) ;
#10833=DIRECTION ( 'NONE',  ( -1.000000000000000000, 0.000000000000000000, 0.000000000000000000 ) ) ;
#10834=VERTEX_POINT ( 'NONE', #18422 ) ;
#10861=CARTESIAN_POINT ( 'NONE',  ( -0.6003936137737501122, 1.122047331090473721, 0.009609423979446465522 ) ) ;
#10882=FACE_OUTER_BOUND ( 'NONE', #12827, .T. ) ;
#10889=( NAMED_UNIT ( * ) SI_UNIT ( $, .STERADIAN. ) SOLID_ANGLE_UNIT ( ) ) ;
#10912=DIRECTION ( 'NONE',  ( 0.000000000000000000, 0.000000000000000000, -1.000000000000000000 ) ) ;
#10959=DIRECTION ( 'NONE',  ( -1.000000000000000000, 0.000000000000000000, 0.000000000000000000 ) ) ;
#11009=ORIENTED_EDGE ( 'NONE', *, *, #13941, .F. ) ;
#11039=CIRCLE ( 'NONE', #25920, 0.1771653543307086520 ) ;
#11080=CARTESIAN_POINT ( 'NONE',  ( -0.1141732283464566844, 0.5570866141732283561, 0.000000000000000000 ) ) ;
#11081=CARTESIAN_POINT ( 'NONE',  ( -0.4055118110236220486, -0.4724409448818898127, 0.9954570744419881656 ) ) ;
#11094=CARTESIAN_POINT ( 'NONE',  ( 1.857656692913385893E-16, 0.000000000000000000, 0.000000000000000000 ) ) ;
#11096=FACE_OUTER_BOUND ( 'NONE', #7467, .T. ) ;
#11124=CARTESIAN_POINT ( 'NONE',  ( -0.4330708661417322913, 0.000000000000000000, 0.000000000000000000 ) ) ;
#11166=EDGE_CURVE ( 'NONE', #13935, #1342, #11847, .T. ) ;
#11172=DIRECTION ( 'NONE',  ( 0.000000000000000000, 0.000000000000000000, -1.000000000000000000 ) ) ;
#11175=CARTESIAN_POINT ( 'NONE',  ( -0.6299212598425196763, -0.4724409448818898127, 0.8182917201112794858 ) ) ;
#11204=CARTESIAN_POINT ( 'NONE',  ( -0.4055118110236220486, -0.4724409448818898127, 0.8182917201112794858 ) ) ;
#11219=DIRECTION ( 'NONE',  ( 1.000000000000000000, 0.000000000000000000, 0.000000000000000000 ) ) ;
#11238=AXIS2_PLACEMENT_3D ( 'NONE', #16089, #15938, #24543 ) ;
#11255=ADVANCED_FACE ( 'NONE', ( #25892 ), #4677, .F. ) ;
#11256=DIRECTION ( 'NONE',  ( -1.000000000000000000, 0.000000000000000000, 0.000000000000000000 ) ) ;
#11265=CARTESIAN_POINT ( 'NONE',  ( -0.5177165354330708347, -0.4724409448818898127, -0.8182917201112815953 ) ) ;
#11268=ORIENTED_EDGE ( 'NONE', *, *, #21213, .F. ) ;
#11275=CIRCLE ( 'NONE', #22162, 0.1771653543307086798 ) ;
#11349=CIRCLE ( 'NONE', #20386, 0.1771653543307086798 ) ;
#11366=DIRECTION ( 'NONE',  ( 0.000000000000000000, 0.000000000000000000, 1.000000000000000000 ) ) ;
#11375=CARTESIAN_POINT ( 'NONE',  ( -0.6299212598425196763, -0.4526313213353582721, 0.9943460912301771426 ) ) ;
#11376=CARTESIAN_POINT ( 'NONE',  ( -0.6299212598425196763, -0.6348133144914134274, 0.8891632684400255782 ) ) ;
#11380=AXIS2_PLACEMENT_3D ( 'NONE', #25117, #7612, #22580 ) ;
#11401=AXIS2_PLACEMENT_3D ( 'NONE', #19116, #10211, #25624 ) ;
#11437=CLOSED_SHELL ( 'NONE', ( #10710, #6575, #25133, #27475, #21815, #6487, #27483, #4397, #7234, #16832, #9544, #18190, #27800, #6281, #25277, #13325, #19806, #11529, #18769, #7339, #11754, #9724, #12785, #23206, #20744, #2956, #13353, #19719, #11473, #18635, #14007, #11541, #20961, #11255, #27709, #8056, #18607 ) ) ;
#11473=ADVANCED_FACE ( 'NONE', ( #12824 ), #24115, .F. ) ;
#11506=FACE_OUTER_BOUND ( 'NONE', #22818, .T. ) ;
#11513=ORIENTED_EDGE ( 'NONE', *, *, #15906, .T. ) ;
#11529=ADVANCED_FACE ( 'NONE', ( #25828 ), #22129, .T. ) ;
#11541=ADVANCED_FACE ( 'NONE', ( #2355 ), #9122, .F. ) ;
#11562=ORIENTED_EDGE ( 'NONE', *, *, #12383, .F. ) ;
#11579=ORIENTED_EDGE ( 'NONE', *, *, #3879, .F. ) ;
#11586=CARTESIAN_POINT ( 'NONE',  ( -0.2066929133858267931, 0.000000000000000000, 0.000000000000000000 ) ) ;
#11587=ORIENTED_EDGE ( 'NONE', *, *, #11780, .T. ) ;
#11588=AXIS2_PLACEMENT_3D ( 'NONE', #5229, #3665, #7923 ) ;
#11616=DIRECTION ( 'NONE',  ( 1.000000000000000000, 0.000000000000000000, 0.000000000000000000 ) ) ;
#11630=CYLINDRICAL_SURFACE ( 'NONE', #10666, 0.1308464566929133932 ) ;
#11650=ORIENTED_EDGE ( 'NONE', *, *, #4311, .F. ) ;
#11676=DIRECTION ( 'NONE',  ( 0.000000000000000000, 1.000000000000000000, 0.000000000000000000 ) ) ;
#11684=CIRCLE ( 'NONE', #24770, 0.6299212598425196763 ) ;
#11708=B_SPLINE_CURVE_WITH_KNOTS ( 'NONE', 3,
 ( #14905, #27746, #25616, #1740, #4009, #12621, #6141, #21240, #10202, #18820, #22941, #27457, #14773, #3862, #10351, #1881, #8390, #10628 ),
 .UNSPECIFIED., .F., .F.,
 ( 4, 2, 2, 2, 2, 2, 2, 2, 4 ),
 ( 0.000000000000000000, 0.2275410946285671421, 0.3413116419428502413, 0.4550821892571332850, 0.5688527365714163286, 0.6826232838856994833, 0.7395085575428416158, 0.7963938311999838593, 0.9101643785142677912 ),
 .UNSPECIFIED. ) ;
#11733=EDGE_CURVE ( 'NONE', #3772, #9494, #20328, .T. ) ;
#11743=AXIS2_PLACEMENT_3D ( 'NONE', #11124, #8454, #13240 ) ;
#11749=CARTESIAN_POINT ( 'NONE',  ( -0.5177165354330708347, -0.4724409448818898127, 0.8182917201112794858 ) ) ;
#11754=ADVANCED_FACE ( 'NONE', ( #18426 ), #13112, .T. ) ;
#11757=CARTESIAN_POINT ( 'NONE',  ( -0.6299212598425196763, 0.9448818897637796255, -9.561468503937007847E-18 ) ) ;
#11766=CARTESIAN_POINT ( 'NONE',  ( -0.6299212598425196763, -0.4724409448818898127, -0.8182917201112815953 ) ) ;
#11778=CARTESIAN_POINT ( 'NONE',  ( 1.877524803149606209E-16, 0.3149606299212598381, 0.000000000000000000 ) ) ;
#11780=EDGE_CURVE ( 'NONE', #26494, #15892, #12648, .T. ) ;
#11800=CARTESIAN_POINT ( 'NONE',  ( -0.6029884523518272976, 1.118955382540533838, -0.03814816047821503742 ) ) ;
#11839=( LENGTH_UNIT ( ) NAMED_UNIT ( * ) SI_UNIT ( $, .METRE. ) ) ;
#11841=PLANE ( 'NONE',  #11238 ) ;
#11847=CIRCLE ( 'NONE', #24030, 0.1771653543307086798 ) ;
#11848=AXIS2_PLACEMENT_3D ( 'NONE', #8932, #6551, #23927 ) ;
#11873=CIRCLE ( 'NONE', #5085, 1.131889763779527547 ) ;
#11885=CONICAL_SURFACE ( 'NONE', #27691, 0.4724409448818898127, 0.7853981625000003852 ) ;
#11922=CIRCLE ( 'NONE', #13721, 0.5118110236220472231 ) ;
#11954=DIRECTION ( 'NONE',  ( 1.000000000000000000, 0.000000000000000000, 0.000000000000000000 ) ) ;
#11962=CIRCLE ( 'NONE', #9232, 0.4330708661417322913 ) ;
#11980=CIRCLE ( 'NONE', #22337, 0.1771653543307086798 ) ;
#11982=VERTEX_POINT ( 'NONE', #7238 ) ;
#12016=ORIENTED_EDGE ( 'NONE', *, *, #16537, .T. ) ;
#12058=EDGE_CURVE ( 'NONE', #2317, #5784, #23044, .T. ) ;
#12093=CARTESIAN_POINT ( 'NONE',  ( -0.6299212598425196763, 1.087444635826771533, 0.1051828227901515783 ) ) ;
#12099=DIRECTION ( 'NONE',  ( 0.000000000000000000, 0.000000000000000000, 1.000000000000000000 ) ) ;
#12150=LINE ( 'NONE', #25437, #1283 ) ;
#12184=DIRECTION ( 'NONE',  ( 1.000000000000000000, 0.000000000000000000, 0.000000000000000000 ) ) ;
#12240=FACE_OUTER_BOUND ( 'NONE', #22302, .T. ) ;
#12288=ORIENTED_EDGE ( 'NONE', *, *, #12663, .F. ) ;
#12305=VERTEX_POINT ( 'NONE', #21847 ) ;
#12331=DIRECTION ( 'NONE',  ( 1.000000000000000000, 0.000000000000000000, 0.000000000000000000 ) ) ;
#12347=EDGE_CURVE ( 'NONE', #24512, #15164, #19129, .T. ) ;
#12371=DIRECTION ( 'NONE',  ( -1.000000000000000000, 0.000000000000000000, 0.000000000000000000 ) ) ;
#12383=EDGE_CURVE ( 'NONE', #4894, #10695, #9377, .T. ) ;
#12409=ORIENTED_EDGE ( 'NONE', *, *, #4311, .T. ) ;
#12412=DIRECTION ( 'NONE',  ( 1.000000000000000000, 0.000000000000000000, 0.000000000000000000 ) ) ;
#12473=CARTESIAN_POINT ( 'NONE',  ( -0.6299212598425196763, -0.4526313213353582721, 0.9943460912301771426 ) ) ;
#12487=AXIS2_PLACEMENT_3D ( 'NONE', #5566, #26741, #7395 ) ;
#12517=DIRECTION ( 'NONE',  ( -1.000000000000000000, 0.000000000000000000, 0.000000000000000000 ) ) ;
#12527=CARTESIAN_POINT ( 'NONE',  ( 1.857656692913385893E-16, 0.000000000000000000, 0.000000000000000000 ) ) ;
#12528=VECTOR ( 'NONE', #6452, 39.37007874015748143 ) ;
#12565=CARTESIAN_POINT ( 'NONE',  ( -0.2362204724409449064, 0.000000000000000000, 0.000000000000000000 ) ) ;
#12573=LINE ( 'NONE', #25845, #12842 ) ;
#12621=CARTESIAN_POINT ( 'NONE',  ( -0.6020310366335483998, -0.5839878592438488836, -0.9562163583985735515 ) ) ;
#12634=EDGE_CURVE ( 'NONE', #19774, #24768, #11349, .T. ) ;
#12643=CARTESIAN_POINT ( 'NONE',  ( -0.6138529921540000212, -0.4891471943186955773, 0.9948696824541676254 ) ) ;
#12648=CIRCLE ( 'NONE', #936, 0.6299212598425196763 ) ;
#12657=DIRECTION ( 'NONE',  ( -1.000000000000000000, 0.000000000000000000, 0.000000000000000000 ) ) ;
#12663=EDGE_CURVE ( 'NONE', #8364, #9929, #2306, .T. ) ;
#12709=ORIENTED_EDGE ( 'NONE', *, *, #12347, .F. ) ;
#12720=CIRCLE ( 'NONE', #18081, 0.1771653543307086798 ) ;
#12722=LINE ( 'NONE', #2398, #22639 ) ;
#12785=ADVANCED_FACE ( 'NONE', ( #9342 ), #17952, .F. ) ;
#12824=FACE_OUTER_BOUND ( 'NONE', #24726, .T. ) ;
#12827=EDGE_LOOP ( 'NONE', ( #13361, #7758, #19041, #6370 ) ) ;
#12839=CARTESIAN_POINT ( 'NONE',  ( -0.6299212598425196763, -0.4724409448818898127, -0.6411263657805729155 ) ) ;
#12842=VECTOR ( 'NONE', #18918, 39.37007874015748143 ) ;
#12845=CIRCLE ( 'NONE', #2020, 0.1771653543307086520 ) ;
#12864=APPLICATION_CONTEXT ( 'automotive_design' ) ;
#12869=CARTESIAN_POINT ( 'NONE',  ( -0.1771653543307086520, -0.5570866141732283561, 6.822343388950805452E-17 ) ) ;
#12878=ORIENTED_EDGE ( 'NONE', *, *, #23187, .F. ) ;
#12897=CIRCLE ( 'NONE', #16961, 0.1308464566929133932 ) ;
#12937=AXIS2_PLACEMENT_3D ( 'NONE', #17382, #192, #15283 ) ;
#12956=VERTEX_POINT ( 'NONE', #5070 ) ;
#12965=DIRECTION ( 'NONE',  ( 0.000000000000000000, 0.000000000000000000, 1.000000000000000000 ) ) ;
#13000=DIRECTION ( 'NONE',  ( -1.000000000000000000, 0.000000000000000000, 0.000000000000000000 ) ) ;
#13027=AXIS2_PLACEMENT_3D ( 'NONE', #24670, #24820, #22426 ) ;
#13049=CIRCLE ( 'NONE', #22074, 0.1308464566929133932 ) ;
#13055=CARTESIAN_POINT ( 'NONE',  ( -0.4055118110236220486, -0.4724409448818898127, -0.6874452634183682020 ) ) ;
#13063=CONICAL_SURFACE ( 'NONE', #4039, 0.4724409448818898127, 0.7853981625000003852 ) ;
#13067=FACE_OUTER_BOUND ( 'NONE', #14921, .T. ) ;
#13091=ORIENTED_EDGE ( 'NONE', *, *, #15192, .T. ) ;
#13111=EDGE_CURVE ( 'NONE', #17618, #5784, #14815, .T. ) ;
#13112=CONICAL_SURFACE ( 'NONE', #3165, 1.112204724409448842, 0.7853981625000011624 ) ;
#13117=CARTESIAN_POINT ( 'NONE',  ( 2.632951206231566310, -0.4724409448818898127, -0.6874452634183682020 ) ) ;
#13126=AXIS2_PLACEMENT_3D ( 'NONE', #8148, #12517, #21280 ) ;
#13155=VERTEX_POINT ( 'NONE', #15083 ) ;
#13167=DIRECTION ( 'NONE',  ( 1.000000000000000000, 0.000000000000000000, 0.000000000000000000 ) ) ;
#13186=CARTESIAN_POINT ( 'NONE',  ( -0.6071195058918599230, -0.6030950601074016593, 0.9382339938617433317 ) ) ;
#13191=ORIENTED_EDGE ( 'NONE', *, *, #23596, .T. ) ;
#13196=CIRCLE ( 'NONE', #11401, 0.1308464566929133932 ) ;
#13208=DIRECTION ( 'NONE',  ( 0.000000000000000000, 0.000000000000000000, 1.000000000000000000 ) ) ;
#13228=ORIENTED_EDGE ( 'NONE', *, *, #18680, .F. ) ;
#13240=DIRECTION ( 'NONE',  ( 0.000000000000000000, 1.000000000000000000, 0.000000000000000000 ) ) ;
#13258=DIRECTION ( 'NONE',  ( 0.000000000000000000, 1.000000000000000000, 0.000000000000000000 ) ) ;
#13268=FACE_OUTER_BOUND ( 'NONE', #14514, .T. ) ;
#13306=CARTESIAN_POINT ( 'NONE',  ( -0.6299212598425196763, 0.9448818897637796255, -9.561468503937007847E-18 ) ) ;
#13314=PLANE ( 'NONE',  #11848 ) ;
#13325=ADVANCED_FACE ( 'NONE', ( #19817 ), #479, .T. ) ;
#13348=CARTESIAN_POINT ( 'NONE',  ( -0.05118110236220472370, 0.5935039370078740717, 0.000000000000000000 ) ) ;
#13353=ADVANCED_FACE ( 'NONE', ( #7515 ), #14304, .F. ) ;
#13361=ORIENTED_EDGE ( 'NONE', *, *, #2175, .F. ) ;
#13372=ORIENTED_EDGE ( 'NONE', *, *, #18017, .T. ) ;
#13413=DIRECTION ( 'NONE',  ( 0.000000000000000000, 0.000000000000000000, -1.000000000000000000 ) ) ;
#13425=ORIENTED_EDGE ( 'NONE', *, *, #15906, .F. ) ;
#13457=CARTESIAN_POINT ( 'NONE',  ( -0.2362204724409449064, 0.000000000000000000, 0.000000000000000000 ) ) ;
#13461=DIRECTION ( 'NONE',  ( -1.000000000000000000, 0.000000000000000000, 0.000000000000000000 ) ) ;
#13466=ORIENTED_EDGE ( 'NONE', *, *, #8797, .F. ) ;
#13594=CIRCLE ( 'NONE', #26657, 0.4330708661417322913 ) ;
#13612=DIRECTION ( 'NONE',  ( -1.000000000000000000, 0.000000000000000000, 0.000000000000000000 ) ) ;
#13615=ORIENTED_EDGE ( 'NONE', *, *, #2293, .T. ) ;
#13633=EDGE_CURVE ( 'NONE', #12956, #27811, #11873, .T. ) ;
#13652=FACE_OUTER_BOUND ( 'NONE', #8876, .T. ) ;
#13695=VERTEX_POINT ( 'NONE', #7074 ) ;
#13708=CARTESIAN_POINT ( 'NONE',  ( -0.05118110236220472370, -0.6299212598425196763, 7.714310545810098438E-17 ) ) ;
#13721=AXIS2_PLACEMENT_3D ( 'NONE', #8384, #12184, #10196 ) ;
#13739=DIRECTION ( 'NONE',  ( -1.000000000000000000, 0.000000000000000000, 0.000000000000000000 ) ) ;
#13756=ORIENTED_EDGE ( 'NONE', *, *, #15454, .F. ) ;
#13787=DIRECTION ( 'NONE',  ( 0.000000000000000000, 0.000000000000000000, 1.000000000000000000 ) ) ;
#13801=EDGE_CURVE ( 'NONE', #5489, #24837, #6932, .T. ) ;
#13806=PRESENTATION_STYLE_ASSIGNMENT (( #16070 ) ) ;
#13879=CARTESIAN_POINT ( 'NONE',  ( -0.6299212598425196763, 0.9448818897637796255, 0.1771653543307086520 ) ) ;
#13888=( GEOMETRIC_REPRESENTATION_CONTEXT ( 3 ) GLOBAL_UNCERTAINTY_ASSIGNED_CONTEXT ( ( #7344 ) ) GLOBAL_UNIT_ASSIGNED_CONTEXT ( ( #9669, #1098, #10889 ) ) REPRESENTATION_CONTEXT ( 'NONE', 'WORKASPACE' ) ) ;
#13935=VERTEX_POINT ( 'NONE', #12839 ) ;
#13941=EDGE_CURVE ( 'NONE', #3772, #23967, #25135, .T. ) ;
#13943=DIRECTION ( 'NONE',  ( -1.000000000000000000, 0.000000000000000000, 0.000000000000000000 ) ) ;
#13964=CARTESIAN_POINT ( 'NONE',  ( -0.1771653543307086520, 0.000000000000000000, 0.000000000000000000 ) ) ;
#14001=DIRECTION ( 'NONE',  ( 0.000000000000000000, -1.000000000000000000, 0.000000000000000000 ) ) ;
#14007=ADVANCED_FACE ( 'NONE', ( #1827 ), #1080, .T. ) ;
#14069=CARTESIAN_POINT ( 'NONE',  ( -0.6088260560327825033, 1.112071903501499648, -0.05864771439951445287 ) ) ;
#14226=CARTESIAN_POINT ( 'NONE',  ( -0.4055118110236220486, 0.9448818897637796255, 0.1308464566929133654 ) ) ;
#14287=ORIENTED_EDGE ( 'NONE', *, *, #8725, .F. ) ;
#14304=CYLINDRICAL_SURFACE ( 'NONE', #4629, 0.1771653543307086798 ) ;
#14322=ORIENTED_EDGE ( 'NONE', *, *, #25909, .T. ) ;
#14324=ORIENTED_EDGE ( 'NONE', *, *, #25329, .F. ) ;
#14395=ADVANCED_BREP_SHAPE_REPRESENTATION ( 'Front Bearing Cover', ( #3076, #11588 ), #10253 ) ;
#14397=CIRCLE ( 'NONE', #5817, 0.4330708661417322913 ) ;
#14419=ORIENTED_EDGE ( 'NONE', *, *, #16954, .F. ) ;
#14439=DIRECTION ( 'NONE',  ( 0.000000000000000000, 0.000000000000000000, 1.000000000000000000 ) ) ;
#14449=DIRECTION ( 'NONE',  ( 0.000000000000000000, 0.000000000000000000, 1.000000000000000000 ) ) ;
#14450=DIRECTION ( 'NONE',  ( 0.000000000000000000, 0.000000000000000000, 1.000000000000000000 ) ) ;
#14485=CARTESIAN_POINT ( 'NONE',  ( -0.3149606299212598381, 0.000000000000000000, 0.000000000000000000 ) ) ;
#14487=FACE_OUTER_BOUND ( 'NONE', #8451, .T. ) ;
#14497=ORIENTED_EDGE ( 'NONE', *, *, #838, .T. ) ;
#14514=EDGE_LOOP ( 'NONE', ( #23123, #11587, #22975, #21753 ) ) ;
#14528=DIRECTION ( 'NONE',  ( 1.000000000000000000, 0.000000000000000000, 0.000000000000000000 ) ) ;
#14532=CARTESIAN_POINT ( 'NONE',  ( 1.857656692913385893E-16, -6.267877317605309469E-17, -0.5118110235513823048 ) ) ;
#14587=AXIS2_PLACEMENT_3D ( 'NONE', #27466, #14913, #27753 ) ;
#14606=CIRCLE ( 'NONE', #20439, 0.6299212598425196763 ) ;
#14620=ORIENTED_EDGE ( 'NONE', *, *, #24469, .F. ) ;
#14650=EDGE_LOOP ( 'NONE', ( #9966, #10084 ) ) ;
#14681=DIRECTION ( 'NONE',  ( -1.000000000000000000, 0.000000000000000000, 0.000000000000000000 ) ) ;
#14735=ORIENTED_EDGE ( 'NONE', *, *, #12634, .T. ) ;
#14773=CARTESIAN_POINT ( 'NONE',  ( -0.6064065885002177803, -0.5142378326778294095, -0.9905099408302305841 ) ) ;
#14801=EDGE_LOOP ( 'NONE', ( #10138, #13191, #22962, #26342 ) ) ;
#14812=DIRECTION ( 'NONE',  ( -1.000000000000000000, 0.000000000000000000, 0.000000000000000000 ) ) ;
#14815=LINE ( 'NONE', #23825, #3700 ) ;
#14817=AXIS2_PLACEMENT_3D ( 'NONE', #11094, #12657, #4052 ) ;
#14855=CARTESIAN_POINT ( 'NONE',  ( -0.6057854838206414572, 1.115659691807754372, 0.04720470158478681094 ) ) ;
#14858=CARTESIAN_POINT ( 'NONE',  ( -0.6102362204724409711, -1.112204724409448842, 0.000000000000000000 ) ) ;
#14905=CARTESIAN_POINT ( 'NONE',  ( -0.6299212598425196763, -0.6348133144914134274, -0.8891632684400255782 ) ) ;
#14913=DIRECTION ( 'NONE',  ( 1.000000000000000000, 0.000000000000000000, 0.000000000000000000 ) ) ;
#14921=EDGE_LOOP ( 'NONE', ( #14324, #20067, #16162, #5671 ) ) ;
#14928=DIRECTION ( 'NONE',  ( 0.000000000000000000, 0.000000000000000000, -1.000000000000000000 ) ) ;
#14962=VERTEX_POINT ( 'NONE', #17662 ) ;
#14974=ORIENTED_EDGE ( 'NONE', *, *, #13633, .F. ) ;
#14977=DIRECTION ( 'NONE',  ( -1.000000000000000000, 0.000000000000000000, 0.000000000000000000 ) ) ;
#14987=CARTESIAN_POINT ( 'NONE',  ( -0.6204317524930640371, 1.098416878719267187, 0.09031125883760274253 ) ) ;
#15001=ORIENTED_EDGE ( 'NONE', *, *, #27438, .T. ) ;
#15022=ORIENTED_EDGE ( 'NONE', *, *, #8155, .F. ) ;
#15079=CARTESIAN_POINT ( 'NONE',  ( 2.632951206231566310, -0.4724409448818898127, -0.8182917201112815953 ) ) ;
#15083=CARTESIAN_POINT ( 'NONE',  ( 1.857656692913385893E-16, 0.000000000000000000, 0.5118110235513823048 ) ) ;
#15107=ORIENTED_EDGE ( 'NONE', *, *, #27146, .T. ) ;
#15164=VERTEX_POINT ( 'NONE', #16956 ) ;
#15191=VERTEX_POINT ( 'NONE', #8198 ) ;
#15192=EDGE_CURVE ( 'NONE', #9494, #13155, #12573, .T. ) ;
#15202=PRODUCT_DEFINITION_FORMATION_WITH_SPECIFIED_SOURCE ( 'ANY', '', #3691, .NOT_KNOWN. ) ;
#15217=ORIENTED_EDGE ( 'NONE', *, *, #2449, .T. ) ;
#15220=ORIENTED_EDGE ( 'NONE', *, *, #15556, .T. ) ;
#15222=ORIENTED_EDGE ( 'NONE', *, *, #7803, .F. ) ;
#15250=CARTESIAN_POINT ( 'NONE',  ( -0.4055118110236220486, -0.4724409448818898127, -0.8182917201112815953 ) ) ;
#15283=DIRECTION ( 'NONE',  ( 0.000000000000000000, 0.000000000000000000, 1.000000000000000000 ) ) ;
#15347=CARTESIAN_POINT ( 'NONE',  ( -0.6299212598425196763, -0.6348133144914134274, 0.8891632684400255782 ) ) ;
#15416=DIRECTION ( 'NONE',  ( 1.000000000000000000, 0.000000000000000000, 0.000000000000000000 ) ) ;
#15442=ORIENTED_EDGE ( 'NONE', *, *, #2778, .T. ) ;
#15454=EDGE_CURVE ( 'NONE', #12305, #17515, #25144, .T. ) ;
#15455=CARTESIAN_POINT ( 'NONE',  ( -0.03937007874015747977, 0.000000000000000000, 0.000000000000000000 ) ) ;
#15489=DIRECTION ( 'NONE',  ( -1.000000000000000000, 0.000000000000000000, 0.000000000000000000 ) ) ;
#15503=CARTESIAN_POINT ( 'NONE',  ( 2.632951206231566310, 0.9448818897637796255, -9.561468503937007847E-18 ) ) ;
#15517=EDGE_LOOP ( 'NONE', ( #16337, #513, #6866, #2473 ) ) ;
#15518=CARTESIAN_POINT ( 'NONE',  ( -0.3149606299212598381, 0.000000000000000000, 0.000000000000000000 ) ) ;
#15525=CARTESIAN_POINT ( 'NONE',  ( -0.5177165354330708347, 0.9448818897637796255, 0.1771653543307086520 ) ) ;
#15543=DIRECTION ( 'NONE',  ( 0.000000000000000000, 1.000000000000000000, 0.000000000000000000 ) ) ;
#15552=EDGE_CURVE ( 'NONE', #15164, #15630, #6181, .T. ) ;
#15556=EDGE_CURVE ( 'NONE', #158, #24837, #26323, .T. ) ;
#15570=DIRECTION ( 'NONE',  ( 1.000000000000000000, 0.000000000000000000, 0.000000000000000000 ) ) ;
#15600=AXIS2_PLACEMENT_3D ( 'NONE', #13457, #11616, #15857 ) ;
#15621=CARTESIAN_POINT ( 'NONE',  ( -0.4055118110236220486, -0.4724409448818898127, 0.8182917201112794858 ) ) ;
#15630=VERTEX_POINT ( 'NONE', #11376 ) ;
#15662=CARTESIAN_POINT ( 'NONE',  ( -0.2362204724409449064, -0.4724409448818898127, -0.6874452634183682020 ) ) ;
#15688=EDGE_CURVE ( 'NONE', #5827, #24512, #1571, .T. ) ;
#15724=CARTESIAN_POINT ( 'NONE',  ( -0.1771653543307086520, 0.5570866141732283561, 0.000000000000000000 ) ) ;
#15727=EDGE_CURVE ( 'NONE', #8482, #2317, #2414, .T. ) ;
#15739=FACE_OUTER_BOUND ( 'NONE', #19180, .T. ) ;
#15779=DIRECTION ( 'NONE',  ( 0.000000000000000000, 1.000000000000000000, 0.000000000000000000 ) ) ;
#15787=CIRCLE ( 'NONE', #27088, 0.1771653543307086520 ) ;
#15809=ORIENTED_EDGE ( 'NONE', *, *, #7082, .F. ) ;
#15857=DIRECTION ( 'NONE',  ( 0.000000000000000000, 1.000000000000000000, 0.000000000000000000 ) ) ;
#15871=DIRECTION ( 'NONE',  ( 1.000000000000000000, 0.000000000000000000, 0.000000000000000000 ) ) ;
#15892=VERTEX_POINT ( 'NONE', #22361 ) ;
#15902=CARTESIAN_POINT ( 'NONE',  ( -0.5905511811023621549, 1.131889763779527547, 0.000000000000000000 ) ) ;
#15906=EDGE_CURVE ( 'NONE', #8482, #17618, #6130, .T. ) ;
#15938=DIRECTION ( 'NONE',  ( 1.000000000000000000, 0.000000000000000000, 0.000000000000000000 ) ) ;
#16028=DIRECTION ( 'NONE',  ( -1.000000000000000000, 0.000000000000000000, 0.000000000000000000 ) ) ;
#16037=EDGE_CURVE ( 'NONE', #15630, #5827, #11980, .T. ) ;
#16043=EDGE_CURVE ( 'NONE', #26494, #25584, #10485, .T. ) ;
#16045=EDGE_LOOP ( 'NONE', ( #5451, #7646, #5727, #7686, #22033, #4647, #7315, #12016, #16470, #7920, #13466 ) ) ;
#16051=EDGE_LOOP ( 'NONE', ( #8905, #22924 ) ) ;
#16070=SURFACE_STYLE_USAGE ( .BOTH. , #3045 ) ;
#16081=AXIS2_PLACEMENT_3D ( 'NONE', #905, #20387, #24339 ) ;
#16089=CARTESIAN_POINT ( 'NONE',  ( -0.2362204724409449064, 0.8809055118110236116, 0.000000000000000000 ) ) ;
#16137=LINE ( 'NONE', #7510, #5639 ) ;
#16162=ORIENTED_EDGE ( 'NONE', *, *, #23187, .T. ) ;
#16166=CYLINDRICAL_SURFACE ( 'NONE', #12487, 0.6299212598425196763 ) ;
#16192=CARTESIAN_POINT ( 'NONE',  ( -0.6003937007829848183, 1.122047244090071727, 1.315345636034250449E-15 ) ) ;
#16225=DIRECTION ( 'NONE',  ( 0.000000000000000000, 1.000000000000000000, 0.000000000000000000 ) ) ;
#16321=( LENGTH_UNIT ( ) NAMED_UNIT ( * ) SI_UNIT ( $, .METRE. ) ) ;
#16337=ORIENTED_EDGE ( 'NONE', *, *, #767, .T. ) ;
#16338=ORIENTED_EDGE ( 'NONE', *, *, #875, .F. ) ;
#16351=DIRECTION ( 'NONE',  ( 0.000000000000000000, 0.000000000000000000, 1.000000000000000000 ) ) ;
#16407=CARTESIAN_POINT ( 'NONE',  ( -0.03937007874015747977, -0.6299212598425196763, 7.714310545810098438E-17 ) ) ;
#16423=EDGE_CURVE ( 'NONE', #11982, #13935, #23348, .T. ) ;
#16444=DIRECTION ( 'NONE',  ( 0.000000000000000000, 0.000000000000000000, 1.000000000000000000 ) ) ;
#16466=ORIENTED_EDGE ( 'NONE', *, *, #7162, .T. ) ;
#16470=ORIENTED_EDGE ( 'NONE', *, *, #11166, .T. ) ;
#16501=AXIS2_PLACEMENT_3D ( 'NONE', #6710, #13461, #19279 ) ;
#16537=EDGE_CURVE ( 'NONE', #14962, #13935, #11275, .T. ) ;
#16538=DIRECTION ( 'NONE',  ( -1.000000000000000000, 0.000000000000000000, 0.000000000000000000 ) ) ;
#16684=LINE ( 'NONE', #21056, #27458 ) ;
#16701=CIRCLE ( 'NONE', #50, 1.131889763779527547 ) ;
#16757=FACE_OUTER_BOUND ( 'NONE', #6114, .T. ) ;
#16764=AXIS2_PLACEMENT_3D ( 'NONE', #15503, #10833, #17195 ) ;
#16821=DIRECTION ( 'NONE',  ( -1.000000000000000000, 0.000000000000000000, 0.000000000000000000 ) ) ;
#16832=ADVANCED_FACE ( 'NONE', ( #562 ), #24553, .F. ) ;
#16870=CIRCLE ( 'NONE', #7370, 0.5570866141732283561 ) ;
#16874=CARTESIAN_POINT ( 'NONE',  ( -0.6265112766918068399, -0.4592307444201776945, -0.9950886577925649457 ) ) ;
#16881=FILL_AREA_STYLE_COLOUR ( '', #25162 ) ;
#16893=CARTESIAN_POINT ( 'NONE',  ( -0.4055118110236220486, 0.9448818897637796255, -9.561468503937007847E-18 ) ) ;
#16920=CARTESIAN_POINT ( 'NONE',  ( -0.01968503937007873988, 0.6246466694403326469, 7.649715443281581808E-17 ) ) ;
#16923=ORIENTED_EDGE ( 'NONE', *, *, #7983, .F. ) ;
#16954=EDGE_CURVE ( 'NONE', #27811, #12956, #16701, .T. ) ;
#16956=CARTESIAN_POINT ( 'NONE',  ( -0.6205616028481958368, -0.4724399524669597450, 0.9954595399567032210 ) ) ;
#16961=AXIS2_PLACEMENT_3D ( 'NONE', #16893, #18995, #14928 ) ;
#17030=AXIS2_PLACEMENT_3D ( 'NONE', #27139, #5379, #14001 ) ;
#17061=ORIENTED_EDGE ( 'NONE', *, *, #585, .T. ) ;
#17080=DIRECTION ( 'NONE',  ( 0.000000000000000000, 0.000000000000000000, 1.000000000000000000 ) ) ;
#17103=ORIENTED_EDGE ( 'NONE', *, *, #9683, .F. ) ;
#17143=AXIS2_PLACEMENT_3D ( 'NONE', #23412, #12371, #6306 ) ;
#17180=CARTESIAN_POINT ( 'NONE',  ( -0.2362204724409449064, 0.9448818897637796255, -9.561468503937007847E-18 ) ) ;
#17195=DIRECTION ( 'NONE',  ( 0.000000000000000000, 0.000000000000000000, -1.000000000000000000 ) ) ;
#17269=DIRECTION ( 'NONE',  ( 1.000000000000000000, 0.000000000000000000, 0.000000000000000000 ) ) ;
#17273=DIRECTION ( 'NONE',  ( 1.000000000000000000, 0.000000000000000000, 0.000000000000000000 ) ) ;
#17327=AXIS2_PLACEMENT_3D ( 'NONE', #13306, #17273, #14439 ) ;
#17328=VERTEX_POINT ( 'NONE', #4430 ) ;
#17343=AXIS2_PLACEMENT_3D ( 'NONE', #17914, #15570, #11172 ) ;
#17348=DIRECTION ( 'NONE',  ( 1.000000000000000000, 0.000000000000000000, 0.000000000000000000 ) ) ;
#17373=VERTEX_POINT ( 'NONE', #20362 ) ;
#17375=DIRECTION ( 'NONE',  ( 0.000000000000000000, -1.000000000000000000, 0.000000000000000000 ) ) ;
#17382=CARTESIAN_POINT ( 'NONE',  ( 1.877524803149606209E-16, 0.000000000000000000, 0.000000000000000000 ) ) ;
#17386=DIRECTION ( 'NONE',  ( 1.000000000000000000, 0.000000000000000000, 0.000000000000000000 ) ) ;
#17399=DIRECTION ( 'NONE',  ( 0.000000000000000000, 0.000000000000000000, 1.000000000000000000 ) ) ;
#17432=CARTESIAN_POINT ( 'NONE',  ( -0.6145042738822253936, -0.6192718686174618625, 0.9188498711560100229 ) ) ;
#17484=DIRECTION ( 'NONE',  ( -1.000000000000000000, 0.000000000000000000, 0.000000000000000000 ) ) ;
#17515=VERTEX_POINT ( 'NONE', #9033 ) ;
#17580=ORIENTED_EDGE ( 'NONE', *, *, #20606, .F. ) ;
#17613=EDGE_LOOP ( 'NONE', ( #13756, #27661, #21505, #1092, #16338, #25006, #25856 ) ) ;
#17618=VERTEX_POINT ( 'NONE', #10747 ) ;
#17654=CARTESIAN_POINT ( 'NONE',  ( -0.4055118110236220486, -0.4724409448818898127, 0.8182917201112794858 ) ) ;
#17662=CARTESIAN_POINT ( 'NONE',  ( -0.6299212598425196763, -0.4526313213353582721, -0.9943460912301771426 ) ) ;
#17693=CARTESIAN_POINT ( 'NONE',  ( 2.632951206231566310, -0.4724409448818898127, -0.9491381768041949885 ) ) ;
#17697=CARTESIAN_POINT ( 'NONE',  ( -0.6050288667202972093, -0.5969381639782070925, 0.9446416071478749288 ) ) ;
#17738=ORIENTED_EDGE ( 'NONE', *, *, #13111, .T. ) ;
#17739=ORIENTED_EDGE ( 'NONE', *, *, #24056, .F. ) ;
#17741=ORIENTED_EDGE ( 'NONE', *, *, #23315, .F. ) ;
#17752=AXIS2_PLACEMENT_3D ( 'NONE', #10436, #10022, #23602 ) ;
#17799=ORIENTED_EDGE ( 'NONE', *, *, #25329, .T. ) ;
#17914=CARTESIAN_POINT ( 'NONE',  ( -0.4055118110236220486, 0.9448818897637796255, -9.561468503937007847E-18 ) ) ;
#17952=CYLINDRICAL_SURFACE ( 'NONE', #18111, 0.1771653543307086520 ) ;
#17967=CARTESIAN_POINT ( 'NONE',  ( -0.1141732283464566844, -0.5570866141732283561, 6.822343388950805452E-17 ) ) ;
#17974=DIRECTION ( 'NONE',  ( 0.000000000000000000, -1.000000000000000000, 0.000000000000000000 ) ) ;
#17985=EDGE_CURVE ( 'NONE', #7640, #11982, #21135, .T. ) ;
#18017=EDGE_CURVE ( 'NONE', #25955, #1342, #19781, .T. ) ;
#18019=EDGE_CURVE ( 'NONE', #9714, #3172, #14397, .T. ) ;
#18081=AXIS2_PLACEMENT_3D ( 'NONE', #3977, #18357, #14449 ) ;
#18107=PLANE ( 'NONE',  #26477 ) ;
#18111=AXIS2_PLACEMENT_3D ( 'NONE', #26587, #13739, #7241 ) ;
#18123=ORIENTED_EDGE ( 'NONE', *, *, #6805, .F. ) ;
#18127=CARTESIAN_POINT ( 'NONE',  ( -0.6108560151425692641, 1.109681230470063618, -0.06506513713565366397 ) ) ;
#18159=CARTESIAN_POINT ( 'NONE',  ( -0.05118110236220472370, -0.5570866141732283561, 6.822343388950805452E-17 ) ) ;
#18190=ADVANCED_FACE ( 'NONE', ( #7730 ), #27083, .T. ) ;
#18284=DIRECTION ( 'NONE',  ( -1.000000000000000000, 0.000000000000000000, 0.000000000000000000 ) ) ;
#18357=DIRECTION ( 'NONE',  ( -1.000000000000000000, 0.000000000000000000, 0.000000000000000000 ) ) ;
#18398=DIRECTION ( 'NONE',  ( 0.000000000000000000, 1.000000000000000000, 0.000000000000000000 ) ) ;
#18422=CARTESIAN_POINT ( 'NONE',  ( -0.2362204724409449064, -0.4724409448818898127, 0.6874452634183660926 ) ) ;
#18426=FACE_OUTER_BOUND ( 'NONE', #23201, .T. ) ;
#18448=DIRECTION ( 'NONE',  ( 1.000000000000000000, 0.000000000000000000, 0.000000000000000000 ) ) ;
#18501=DIRECTION ( 'NONE',  ( 0.000000000000000000, -1.000000000000000000, 0.000000000000000000 ) ) ;
#18533=VECTOR ( 'NONE', #10668, 39.37007874015748143 ) ;
#18558=EDGE_LOOP ( 'NONE', ( #15222, #21545, #15220, #4058 ) ) ;
#18581=CARTESIAN_POINT ( 'NONE',  ( -0.4055118110236220486, -0.4724409448818898127, -0.8182917201112815953 ) ) ;
#18588=CARTESIAN_POINT ( 'NONE',  ( -0.2362204724409449064, -0.4724409448818898127, 0.8182917201112794858 ) ) ;
#18602=( NAMED_UNIT ( * ) SI_UNIT ( $, .STERADIAN. ) SOLID_ANGLE_UNIT ( ) ) ;
#18607=ADVANCED_FACE ( 'NONE', ( #6781 ), #13063, .F. ) ;
#18635=ADVANCED_FACE ( 'NONE', ( #13268 ), #26258, .T. ) ;
#18680=EDGE_CURVE ( 'NONE', #13695, #10695, #9891, .T. ) ;
#18695=VECTOR ( 'NONE', #19699, 39.37007874015748143 ) ;
#18727=DIRECTION ( 'NONE',  ( 0.000000000000000000, 1.000000000000000000, 0.000000000000000000 ) ) ;
#18769=ADVANCED_FACE ( 'NONE', ( #22872, #5633, #27108, #7613, #1120 ), #11841, .T. ) ;
#18776=EDGE_LOOP ( 'NONE', ( #18974, #17103, #9811, #6152 ) ) ;
#18820=CARTESIAN_POINT ( 'NONE',  ( -0.6016343471712377600, -0.5391005349154589510, -0.9826765462749172952 ) ) ;
#18826=CARTESIAN_POINT ( 'NONE',  ( -0.3149606299212598381, 0.000000000000000000, 0.4330708661417322913 ) ) ;
#18843=ORIENTED_EDGE ( 'NONE', *, *, #10208, .T. ) ;
#18858=PLANE ( 'NONE',  #13126 ) ;
#18914=CARTESIAN_POINT ( 'NONE',  ( -0.1771653543307086520, -0.6299212598425196763, 7.714310545810098438E-17 ) ) ;
#18918=DIRECTION ( 'NONE',  ( 0.7071067818211390632, 0.000000000000000000, 0.7071067805519560823 ) ) ;
#18920=DIRECTION ( 'NONE',  ( 0.7071067818211385081, -0.7071067805519564153, 0.000000000000000000 ) ) ;
#18974=ORIENTED_EDGE ( 'NONE', *, *, #838, .F. ) ;
#18995=DIRECTION ( 'NONE',  ( 1.000000000000000000, 0.000000000000000000, 0.000000000000000000 ) ) ;
#19020=EDGE_LOOP ( 'NONE', ( #18123, #8551, #10094, #15809 ) ) ;
#19041=ORIENTED_EDGE ( 'NONE', *, *, #7983, .T. ) ;
#19042=EDGE_CURVE ( 'NONE', #1699, #9929, #9779, .T. ) ;
#19084=AXIS2_PLACEMENT_3D ( 'NONE', #20073, #9055, #10912 ) ;
#19112=CARTESIAN_POINT ( 'NONE',  ( -0.2362204724409449064, 0.6299212598425196763, 0.000000000000000000 ) ) ;
#19116=CARTESIAN_POINT ( 'NONE',  ( -0.2362204724409449064, -0.4724409448818898127, -0.8182917201112815953 ) ) ;
#19125=CIRCLE ( 'NONE', #17343, 0.1308464566929133932 ) ;
#19126=EDGE_CURVE ( 'NONE', #7494, #24512, #21513, .T. ) ;
#19129=B_SPLINE_CURVE_WITH_KNOTS ( 'NONE', 3,
 ( #11375, #9816, #19995, #7143 ),
 .UNSPECIFIED., .F., .F.,
 ( 4, 4 ),
 ( 0.000000000000000000, 0.08984410251848014284 ),
 .UNSPECIFIED. ) ;
#19134=CARTESIAN_POINT ( 'NONE',  ( -0.6016344796479202728, -0.5390998427281981087, 0.9826767787459085302 ) ) ;
#19161=ORIENTED_EDGE ( 'NONE', *, *, #16954, .T. ) ;
#19180=EDGE_LOOP ( 'NONE', ( #6771, #906 ) ) ;
#19185=EDGE_LOOP ( 'NONE', ( #5246, #14287, #7781, #24714, #15022 ) ) ;
#19276=CARTESIAN_POINT ( 'NONE',  ( -0.1771653543307086520, 0.6299212598425196763, 0.000000000000000000 ) ) ;
#19277=CARTESIAN_POINT ( 'NONE',  ( -0.6064063350436810218, -0.5142385541152183492, 0.9905098495108229928 ) ) ;
#19279=DIRECTION ( 'NONE',  ( 0.000000000000000000, 0.000000000000000000, 1.000000000000000000 ) ) ;
#19294=DIRECTION ( 'NONE',  ( 0.000000000000000000, 0.000000000000000000, -1.000000000000000000 ) ) ;
#19305=EDGE_LOOP ( 'NONE', ( #3884, #12409 ) ) ;
#19343=CARTESIAN_POINT ( 'NONE',  ( -0.6299212598425196763, 1.087444635826771533, 0.1051828227901515783 ) ) ;
#19359=DIRECTION ( 'NONE',  ( 0.000000000000000000, 0.000000000000000000, 1.000000000000000000 ) ) ;
#19461=DIRECTION ( 'NONE',  ( 0.000000000000000000, 0.000000000000000000, 1.000000000000000000 ) ) ;
#19475=CARTESIAN_POINT ( 'NONE',  ( -0.6010422146565906898, 1.121275077793808528, 0.01914631898548286096 ) ) ;
#19497=CYLINDRICAL_SURFACE ( 'NONE', #12937, 0.4330708661417322913 ) ;
#19506=DIRECTION ( 'NONE',  ( 0.000000000000000000, 0.000000000000000000, 1.000000000000000000 ) ) ;
#19515=EDGE_CURVE ( 'NONE', #17328, #4894, #24561, .T. ) ;
#19565=ORIENTED_EDGE ( 'NONE', *, *, #22601, .F. ) ;
#19572=CARTESIAN_POINT ( 'NONE',  ( 2.632951206231566310, -0.4724409448818898127, 0.8182917201112794858 ) ) ;
#19590=AXIS2_PLACEMENT_3D ( 'NONE', #24568, #4945, #20482 ) ;
#19612=DIRECTION ( 'NONE',  ( -1.000000000000000000, 0.000000000000000000, 0.000000000000000000 ) ) ;
#19656=CARTESIAN_POINT ( 'NONE',  ( -0.5177165354330708347, -0.4724409448818898127, 0.8182917201112794858 ) ) ;
#19699=DIRECTION ( 'NONE',  ( 1.000000000000000000, 0.000000000000000000, 0.000000000000000000 ) ) ;
#19704=ORIENTED_EDGE ( 'NONE', *, *, #15552, .F. ) ;
#19719=ADVANCED_FACE ( 'NONE', ( #10658, #4711 ), #26324, .T. ) ;
#19729=VERTEX_POINT ( 'NONE', #24072 ) ;
#19741=ORIENTED_EDGE ( 'NONE', *, *, #272, .T. ) ;
#19748=LINE ( 'NONE', #6348, #52 ) ;
#19766=CARTESIAN_POINT ( 'NONE',  ( -0.02559055118110236185, 0.000000000000000000, 0.000000000000000000 ) ) ;
#19769=CYLINDRICAL_SURFACE ( 'NONE', #7618, 0.1771653543307086798 ) ;
#19774=VERTEX_POINT ( 'NONE', #11081 ) ;
#19781=CIRCLE ( 'NONE', #26533, 1.092519685039370136 ) ;
#19806=ADVANCED_FACE ( 'NONE', ( #19968, #15739 ), #2850, .T. ) ;
#19814=CARTESIAN_POINT ( 'NONE',  ( -0.2362204724409449064, -0.4724409448818898127, 0.8182917201112794858 ) ) ;
#19817=FACE_OUTER_BOUND ( 'NONE', #18558, .T. ) ;
#19830=CARTESIAN_POINT ( 'NONE',  ( -0.6010692214156458935, -0.5770957586667881944, 0.9615147744183358824 ) ) ;
#19862=FACE_OUTER_BOUND ( 'NONE', #27634, .T. ) ;
#19874=VERTEX_POINT ( 'NONE', #24465 ) ;
#19950=DIRECTION ( 'NONE',  ( 0.000000000000000000, 0.000000000000000000, -1.000000000000000000 ) ) ;
#19968=FACE_BOUND ( 'NONE', #26241, .T. ) ;
#19984=CARTESIAN_POINT ( 'NONE',  ( 1.877524803149606209E-16, 0.000000000000000000, 0.000000000000000000 ) ) ;
#19988=AXIS2_PLACEMENT_3D ( 'NONE', #15518, #11256, #19461 ) ;
#19995=CARTESIAN_POINT ( 'NONE',  ( -0.6233905297002754198, -0.4658379333990866900, 0.9954608945794582997 ) ) ;
#20035=DIRECTION ( 'NONE',  ( 1.000000000000000000, 0.000000000000000000, 0.000000000000000000 ) ) ;
#20041=DIRECTION ( 'NONE',  ( 0.000000000000000000, 0.000000000000000000, -1.000000000000000000 ) ) ;
#20067=ORIENTED_EDGE ( 'NONE', *, *, #5984, .F. ) ;
#20073=CARTESIAN_POINT ( 'NONE',  ( 2.632951206231566310, -0.4724409448818898127, -0.8182917201112815953 ) ) ;
#20082=CARTESIAN_POINT ( 'NONE',  ( -0.4055118110236220486, -0.4724409448818898127, -0.9491381768041949885 ) ) ;
#20087=VECTOR ( 'NONE', #1382, 39.37007874015748143 ) ;
#20090=CARTESIAN_POINT ( 'NONE',  ( -0.4055118110236220486, 0.9448818897637796255, -9.561468503937007847E-18 ) ) ;
#20123=ORIENTED_EDGE ( 'NONE', *, *, #8900, .F. ) ;
#20168=( NAMED_UNIT ( * ) PLANE_ANGLE_UNIT ( ) SI_UNIT ( $, .RADIAN. ) ) ;
#20257=CARTESIAN_POINT ( 'NONE',  ( -0.3149606299212598381, 5.303588500244442984E-17, -0.4330708661417322913 ) ) ;
#20278=AXIS2_PLACEMENT_3D ( 'NONE', #19984, #9369, #13208 ) ;
#20287=CARTESIAN_POINT ( 'NONE',  ( -0.5177165354330708347, -0.4724409448818898127, -0.8182917201112815953 ) ) ;
#20299=VECTOR ( 'NONE', #17484, 39.37007874015748143 ) ;
#20328=CIRCLE ( 'NONE', #27564, 0.4330708661417322913 ) ;
#20362=CARTESIAN_POINT ( 'NONE',  ( -0.4055118110236220486, -0.4724409448818898127, 0.9491381768041928790 ) ) ;
#20381=DIRECTION ( 'NONE',  ( 1.000000000000000000, 0.000000000000000000, 0.000000000000000000 ) ) ;
#20386=AXIS2_PLACEMENT_3D ( 'NONE', #11204, #4304, #21678 ) ;
#20387=DIRECTION ( 'NONE',  ( 1.000000000000000000, 0.000000000000000000, 0.000000000000000000 ) ) ;
#20388=DIRECTION ( 'NONE',  ( 1.000000000000000000, 0.000000000000000000, 0.000000000000000000 ) ) ;
#20397=DIRECTION ( 'NONE',  ( 1.000000000000000000, 0.000000000000000000, 0.000000000000000000 ) ) ;
#20439=AXIS2_PLACEMENT_3D ( 'NONE', #15455, #13167, #21942 ) ;
#20482=DIRECTION ( 'NONE',  ( 0.000000000000000000, -1.000000000000000000, 0.000000000000000000 ) ) ;
#20539=CARTESIAN_POINT ( 'NONE',  ( -0.4330708661417322913, 1.131889763779527547, 0.000000000000000000 ) ) ;
#20578=EDGE_CURVE ( 'NONE', #19729, #25584, #16684, .T. ) ;
#20582=DIRECTION ( 'NONE',  ( 1.000000000000000000, 0.000000000000000000, 0.000000000000000000 ) ) ;
#20591=CARTESIAN_POINT ( 'NONE',  ( -0.4055118110236220486, -0.4724409448818898127, -0.8182917201112815953 ) ) ;
#20598=ORIENTED_EDGE ( 'NONE', *, *, #15688, .F. ) ;
#20606=EDGE_CURVE ( 'NONE', #15892, #25182, #12150, .T. ) ;
#20624=DIRECTION ( 'NONE',  ( 0.000000000000000000, 1.000000000000000000, 0.000000000000000000 ) ) ;
#20631=CARTESIAN_POINT ( 'NONE',  ( -0.5177165354330708347, 0.9448818897637796255, -0.1771653543307086520 ) ) ;
#20664=ORIENTED_EDGE ( 'NONE', *, *, #767, .F. ) ;
#20677=CARTESIAN_POINT ( 'NONE',  ( -0.2362204724409449064, -0.4724409448818898127, -0.9491381768041949885 ) ) ;
#20681=DIRECTION ( 'NONE',  ( 0.000000000000000000, -1.000000000000000000, 0.000000000000000000 ) ) ;
#20744=ADVANCED_FACE ( 'NONE', ( #7288 ), #19769, .F. ) ;
#20760=VERTEX_POINT ( 'NONE', #14226 ) ;
#20792=VECTOR ( 'NONE', #3162, 39.37007874015748854 ) ;
#20801=VERTEX_POINT ( 'NONE', #26778 ) ;
#20861=CARTESIAN_POINT ( 'NONE',  ( -0.07874015748031495954, 5.303588500244442984E-17, -0.4330708661417322913 ) ) ;
#20873=ORIENTED_EDGE ( 'NONE', *, *, #24629, .T. ) ;
#20961=ADVANCED_FACE ( 'NONE', ( #13067 ), #2319, .F. ) ;
#20997=AXIS2_PLACEMENT_3D ( 'NONE', #22803, #17386, #20681 ) ;
#21051=ORIENTED_EDGE ( 'NONE', *, *, #2175, .T. ) ;
#21053=CARTESIAN_POINT ( 'NONE',  ( -0.2362204724409449064, 0.9448818897637796255, -0.1308464566929134210 ) ) ;
#21056=CARTESIAN_POINT ( 'NONE',  ( -0.01968503937007873988, -0.6246466694403326469, 0.000000000000000000 ) ) ;
#21135=CIRCLE ( 'NONE', #7152, 0.1771653543307086798 ) ;
#21145=B_SPLINE_CURVE_WITH_KNOTS ( 'NONE', 3,
 ( #2241, #10861, #19475, #172, #6222, #14855, #23331, #23469, #10730, #14987, #19343 ),
 .UNSPECIFIED., .F., .F.,
 ( 4, 2, 1, 2, 2, 4 ),
 ( 0.5000000000000000000, 0.6249999999999993339, 0.6874999999999988898, 0.7187499999999990008, 0.7499999999999991118, 1.000000000000000000 ),
 .UNSPECIFIED. ) ;
#21151=DIRECTION ( 'NONE',  ( 0.000000000000000000, 0.000000000000000000, -1.000000000000000000 ) ) ;
#21213=EDGE_CURVE ( 'NONE', #1342, #15191, #11708, .T. ) ;
#21240=CARTESIAN_POINT ( 'NONE',  ( -0.6002207073317223918, -0.5625436374629609881, -0.9710811323272637852 ) ) ;
#21270=CARTESIAN_POINT ( 'NONE',  ( -0.6098674607377709833, -0.5016125552355906736, 0.9930863283251144535 ) ) ;
#21280=DIRECTION ( 'NONE',  ( 0.000000000000000000, 0.000000000000000000, 1.000000000000000000 ) ) ;
#21342=AXIS2_PLACEMENT_3D ( 'NONE', #15621, #24085, #6998 ) ;
#21352=DIRECTION ( 'NONE',  ( 1.000000000000000000, 0.000000000000000000, 0.000000000000000000 ) ) ;
#21355=FACE_OUTER_BOUND ( 'NONE', #23104, .T. ) ;
#21435=SHAPE_DEFINITION_REPRESENTATION ( #24888, #24703 ) ;
#21445=EDGE_LOOP ( 'NONE', ( #20123, #5519, #22114, #12709, #20598 ) ) ;
#21458=EDGE_LOOP ( 'NONE', ( #6813, #1711 ) ) ;
#21463=DIRECTION ( 'NONE',  ( 0.000000000000000000, -1.000000000000000000, 0.000000000000000000 ) ) ;
#21505=ORIENTED_EDGE ( 'NONE', *, *, #7082, .T. ) ;
#21513=CIRCLE ( 'NONE', #9298, 1.092519685039370136 ) ;
#21519=ORIENTED_EDGE ( 'NONE', *, *, #6214, .F. ) ;
#21542=CIRCLE ( 'NONE', #26053, 0.1308464566929133932 ) ;
#21545=ORIENTED_EDGE ( 'NONE', *, *, #2149, .T. ) ;
#21586=EDGE_LOOP ( 'NONE', ( #11513, #17738, #392, #26523 ) ) ;
#21611=DIRECTION ( 'NONE',  ( -1.000000000000000000, 0.000000000000000000, 0.000000000000000000 ) ) ;
#21678=DIRECTION ( 'NONE',  ( 0.000000000000000000, 0.000000000000000000, 1.000000000000000000 ) ) ;
#21737=DIRECTION ( 'NONE',  ( -1.000000000000000000, 0.000000000000000000, 0.000000000000000000 ) ) ;
#21753=ORIENTED_EDGE ( 'NONE', *, *, #25951, .F. ) ;
#21815=ADVANCED_FACE ( 'NONE', ( #19862 ), #2341, .F. ) ;
#21835=FACE_OUTER_BOUND ( 'NONE', #21458, .T. ) ;
#21843=ORIENTED_EDGE ( 'NONE', *, *, #16043, .T. ) ;
#21847=CARTESIAN_POINT ( 'NONE',  ( -0.4055118110236220486, 0.9448818897637796255, -0.1771653543307086520 ) ) ;
#21899=DIMENSIONAL_EXPONENTS ( 1.000000000000000000, 0.000000000000000000, 0.000000000000000000, 0.000000000000000000, 0.000000000000000000, 0.000000000000000000, 0.000000000000000000 ) ;
#21904=CARTESIAN_POINT ( 'NONE',  ( -0.6233907401648717261, -0.4658374228745700285, -0.9954608982700638986 ) ) ;
#21909=VECTOR ( 'NONE', #12331, 39.37007874015748143 ) ;
#21942=DIRECTION ( 'NONE',  ( 0.000000000000000000, -1.000000000000000000, 0.000000000000000000 ) ) ;
#21959=DIRECTION ( 'NONE',  ( 0.000000000000000000, -1.000000000000000000, 0.000000000000000000 ) ) ;
#21998=DIRECTION ( 'NONE',  ( 0.000000000000000000, 1.000000000000000000, 0.000000000000000000 ) ) ;
#22008=EDGE_LOOP ( 'NONE', ( #1485, #21843, #8652, #17580 ) ) ;
#22033=ORIENTED_EDGE ( 'NONE', *, *, #25062, .T. ) ;
#22039=CIRCLE ( 'NONE', #9854, 0.1308464566929133932 ) ;
#22043=DIRECTION ( 'NONE',  ( 1.000000000000000000, 0.000000000000000000, 0.000000000000000000 ) ) ;
#22074=AXIS2_PLACEMENT_3D ( 'NONE', #18588, #14681, #21151 ) ;
#22078=ORIENTED_EDGE ( 'NONE', *, *, #2778, .F. ) ;
#22114=ORIENTED_EDGE ( 'NONE', *, *, #8421, .T. ) ;
#22127=EDGE_LOOP ( 'NONE', ( #23642, #6821 ) ) ;
#22129=CYLINDRICAL_SURFACE ( 'NONE', #25407, 0.6299212598425196763 ) ;
#22162=AXIS2_PLACEMENT_3D ( 'NONE', #190, #441, #19359 ) ;
#22170=CARTESIAN_POINT ( 'NONE',  ( -0.4055118110236220486, 0.9448818897637796255, -9.561468503937007847E-18 ) ) ;
#22188=AXIS2_PLACEMENT_3D ( 'NONE', #9904, #1570, #18501 ) ;
#22302=EDGE_LOOP ( 'NONE', ( #25442, #3289, #19565, #7566 ) ) ;
#22337=AXIS2_PLACEMENT_3D ( 'NONE', #23081, #6269, #1877 ) ;
#22361=CARTESIAN_POINT ( 'NONE',  ( -0.05118110236220472370, 0.6299212598425196763, 0.000000000000000000 ) ) ;
#22376=DIRECTION ( 'NONE',  ( 0.000000000000000000, 1.000000000000000000, 0.000000000000000000 ) ) ;
#22402=CARTESIAN_POINT ( 'NONE',  ( -0.6155566689407767633, 1.104160307814390229, -0.07772139087775030430 ) ) ;
#22410=DIRECTION ( 'NONE',  ( 0.000000000000000000, -1.000000000000000000, 0.000000000000000000 ) ) ;
#22426=DIRECTION ( 'NONE',  ( 0.000000000000000000, 1.000000000000000000, 0.000000000000000000 ) ) ;
#22520=FACE_BOUND ( 'NONE', #8304, .T. ) ;
#22524=CIRCLE ( 'NONE', #25678, 0.1308464566929133932 ) ;
#22536=CARTESIAN_POINT ( 'NONE',  ( -0.6102362204724409711, 1.112204724409448842, -1.362057955744595713E-16 ) ) ;
#22580=DIRECTION ( 'NONE',  ( 0.000000000000000000, 0.000000000000000000, -1.000000000000000000 ) ) ;
#22598=DIRECTION ( 'NONE',  ( 1.000000000000000000, 0.000000000000000000, 0.000000000000000000 ) ) ;
#22601=EDGE_CURVE ( 'NONE', #24837, #5489, #16870, .T. ) ;
#22622=VECTOR ( 'NONE', #3561, 39.37007874015748143 ) ;
#22639=VECTOR ( 'NONE', #13000, 39.37007874015748143 ) ;
#22658=LINE ( 'NONE', #7971, #951 ) ;
#22681=CARTESIAN_POINT ( 'NONE',  ( -0.6003938747882047178, 1.122047070076019004, -0.01921884795888584296 ) ) ;
#22700=AXIS2_PLACEMENT_3D ( 'NONE', #23200, #16538, #14450 ) ;
#22803=CARTESIAN_POINT ( 'NONE',  ( -0.03937007874015747977, 0.000000000000000000, 0.000000000000000000 ) ) ;
#22818=EDGE_LOOP ( 'NONE', ( #4284, #7659 ) ) ;
#22872=FACE_BOUND ( 'NONE', #8357, .T. ) ;
#22877=ORIENTED_EDGE ( 'NONE', *, *, #2720, .F. ) ;
#22924=ORIENTED_EDGE ( 'NONE', *, *, #9315, .T. ) ;
#22941=CARTESIAN_POINT ( 'NONE',  ( -0.6028220648874946797, -0.5309697779843188803, -0.9857434533500031293 ) ) ;
#22962=ORIENTED_EDGE ( 'NONE', *, *, #15727, .T. ) ;
#22975=ORIENTED_EDGE ( 'NONE', *, *, #20606, .T. ) ;
#22989=CARTESIAN_POINT ( 'NONE',  ( -0.4330708661417322913, 0.000000000000000000, 0.000000000000000000 ) ) ;
#23009=ORIENTED_EDGE ( 'NONE', *, *, #585, .F. ) ;
#23043=ORIENTED_EDGE ( 'NONE', *, *, #416, .T. ) ;
#23044=CIRCLE ( 'NONE', #480, 0.6299212598425196763 ) ;
#23051=DIRECTION ( 'NONE',  ( -1.000000000000000000, 0.000000000000000000, 0.000000000000000000 ) ) ;
#23081=CARTESIAN_POINT ( 'NONE',  ( -0.6299212598425196763, -0.4724409448818898127, 0.8182917201112794858 ) ) ;
#23104=EDGE_LOOP ( 'NONE', ( #27350, #7061, #2635, #19704, #10648 ) ) ;
#23123=ORIENTED_EDGE ( 'NONE', *, *, #16043, .F. ) ;
#23138=CONICAL_SURFACE ( 'NONE', #14587, 1.112204724409448842, 0.7853981625000011624 ) ;
#23187=EDGE_CURVE ( 'NONE', #10834, #26561, #25228, .T. ) ;
#23199=AXIS2_PLACEMENT_3D ( 'NONE', #27440, #9915, #27163 ) ;
#23200=CARTESIAN_POINT ( 'NONE',  ( -0.4055118110236220486, -0.4724409448818898127, 0.8182917201112794858 ) ) ;
#23201=EDGE_LOOP ( 'NONE', ( #11562, #8269, #3176, #27441, #1976, #2618, #23289, #8538 ) ) ;
#23206=ADVANCED_FACE ( 'NONE', ( #5895, #16757 ), #18858, .T. ) ;
#23289=ORIENTED_EDGE ( 'NONE', *, *, #6214, .T. ) ;
#23315=EDGE_CURVE ( 'NONE', #26561, #17373, #4897, .T. ) ;
#23331=CARTESIAN_POINT ( 'NONE',  ( -0.6069206441216355996, 1.114319256831733274, 0.05180297602608902041 ) ) ;
#23342=VECTOR ( 'NONE', #12412, 39.37007874015748143 ) ;
#23348=LINE ( 'NONE', #27569, #918 ) ;
#23365=DIRECTION ( 'NONE',  ( -1.000000000000000000, 0.000000000000000000, 0.000000000000000000 ) ) ;
#23391=ORIENTED_EDGE ( 'NONE', *, *, #11166, .F. ) ;
#23399=CARTESIAN_POINT ( 'NONE',  ( -0.6169740991250696194, -0.4807978361619021923, 0.9954634121926729806 ) ) ;
#23412=CARTESIAN_POINT ( 'NONE',  ( -0.5177165354330708347, 0.9448818897637796255, -9.561468503937007847E-18 ) ) ;
#23424=DIRECTION ( 'NONE',  ( 1.000000000000000000, 0.000000000000000000, 0.000000000000000000 ) ) ;
#23454=FACE_OUTER_BOUND ( 'NONE', #25554, .T. ) ;
#23461=VECTOR ( 'NONE', #4564, 39.37007874015748143 ) ;
#23469=CARTESIAN_POINT ( 'NONE',  ( -0.6075516362842373619, 1.113574658101797121, 0.05417226358486029736 ) ) ;
#23473=VERTEX_POINT ( 'NONE', #12869 ) ;
#23500=EDGE_LOOP ( 'NONE', ( #25709, #27212, #4815, #24225 ) ) ;
#23561=VECTOR ( 'NONE', #6426, 39.37007874015748143 ) ;
#23596=EDGE_CURVE ( 'NONE', #17618, #8482, #10081, .T. ) ;
#23602=DIRECTION ( 'NONE',  ( 0.000000000000000000, -1.000000000000000000, 0.000000000000000000 ) ) ;
#23642=ORIENTED_EDGE ( 'NONE', *, *, #9683, .T. ) ;
#23659=FACE_OUTER_BOUND ( 'NONE', #16045, .T. ) ;
#23718=VECTOR ( 'NONE', #17269, 39.37007874015748143 ) ;
#23825=CARTESIAN_POINT ( 'NONE',  ( -0.2066929133858267931, -0.6299212598425196763, 7.714310545810098438E-17 ) ) ;
#23857=CARTESIAN_POINT ( 'NONE',  ( 2.632951206231566310, 0.9448818897637796255, -9.561468503937007847E-18 ) ) ;
#23862=CYLINDRICAL_SURFACE ( 'NONE', #11743, 1.131889763779527547 ) ;
#23927=DIRECTION ( 'NONE',  ( 0.000000000000000000, 0.000000000000000000, 1.000000000000000000 ) ) ;
#23967=VERTEX_POINT ( 'NONE', #14532 ) ;
#24030=AXIS2_PLACEMENT_3D ( 'NONE', #11766, #20388, #1046 ) ;
#24056=EDGE_CURVE ( 'NONE', #10695, #13695, #4671, .T. ) ;
#24072=CARTESIAN_POINT ( 'NONE',  ( 1.857656692913385893E-16, -0.6193720790381457286, 0.000000000000000000 ) ) ;
#24085=DIRECTION ( 'NONE',  ( 1.000000000000000000, 0.000000000000000000, 0.000000000000000000 ) ) ;
#24115=PLANE ( 'NONE',  #19988 ) ;
#24136=AXIS2_PLACEMENT_3D ( 'NONE', #11175, #26286, #17399 ) ;
#24152=AXIS2_PLACEMENT_3D ( 'NONE', #11757, #20381, #1039 ) ;
#24163=CARTESIAN_POINT ( 'NONE',  ( -0.2362204724409449064, 0.000000000000000000, 0.000000000000000000 ) ) ;
#24199=VECTOR ( 'NONE', #15871, 39.37007874015748143 ) ;
#24222=CARTESIAN_POINT ( 'NONE',  ( -0.4055118110236220486, -0.4724409448818898127, -0.8182917201112815953 ) ) ;
#24225=ORIENTED_EDGE ( 'NONE', *, *, #25951, .T. ) ;
#24298=EDGE_CURVE ( 'NONE', #17515, #17328, #10099, .T. ) ;
#24306=VECTOR ( 'NONE', #18920, 39.37007874015748854 ) ;
#24320=ORIENTED_EDGE ( 'NONE', *, *, #11733, .F. ) ;
#24339=DIRECTION ( 'NONE',  ( 0.000000000000000000, 1.000000000000000000, 0.000000000000000000 ) ) ;
#24464=PRODUCT_DEFINITION ( 'UNKNOWN', '', #15202, #3157 ) ;
#24465=CARTESIAN_POINT ( 'NONE',  ( -0.2362204724409449064, -0.4724409448818898127, 0.9491381768041928790 ) ) ;
#24469=EDGE_CURVE ( 'NONE', #23967, #13155, #11922, .T. ) ;
#24477=CARTESIAN_POINT ( 'NONE',  ( 2.632951206231566310, -0.4724409448818898127, 0.8182917201112794858 ) ) ;
#24506=CARTESIAN_POINT ( 'NONE',  ( -0.6251768273491621342, 1.092930385926066394, -0.09774754414306212336 ) ) ;
#24512=VERTEX_POINT ( 'NONE', #12473 ) ;
#24513=DIRECTION ( 'NONE',  ( 1.000000000000000000, 0.000000000000000000, 0.000000000000000000 ) ) ;
#24521=CIRCLE ( 'NONE', #23199, 0.1308464566929133932 ) ;
#24543=DIRECTION ( 'NONE',  ( 0.000000000000000000, 1.000000000000000000, 0.000000000000000000 ) ) ;
#24553=CYLINDRICAL_SURFACE ( 'NONE', #17143, 0.1771653543307086520 ) ;
#24561=B_SPLINE_CURVE_WITH_KNOTS ( 'NONE', 3,
 ( #939, #24506, #5156, #22402, #5303, #18127, #7418, #14069, #11800, #22681, #16192 ),
 .UNSPECIFIED., .F., .F.,
 ( 4, 2, 1, 2, 2, 4 ),
 ( 0.000000000000000000, 0.1250000000000002220, 0.1875000000000006661, 0.2187500000000006384, 0.2500000000000006106, 0.5000000000000000000 ),
 .UNSPECIFIED. ) ;
#24568=CARTESIAN_POINT ( 'NONE',  ( -0.5905511811023621549, 0.000000000000000000, 0.000000000000000000 ) ) ;
#24576=DIRECTION ( 'NONE',  ( 1.000000000000000000, 0.000000000000000000, 0.000000000000000000 ) ) ;
#24629=EDGE_CURVE ( 'NONE', #4795, #12305, #11039, .T. ) ;
#24670=CARTESIAN_POINT ( 'NONE',  ( -0.05118110236220472370, 0.000000000000000000, 0.000000000000000000 ) ) ;
#24681=( CONVERSION_BASED_UNIT ( 'INCH', #9419 ) LENGTH_UNIT ( ) NAMED_UNIT ( #21899 ) ) ;
#24703=SHAPE_REPRESENTATION ( 'Front Bearing Cover', ( #11588 ), #10253 ) ;
#24714=ORIENTED_EDGE ( 'NONE', *, *, #16537, .F. ) ;
#24726=EDGE_LOOP ( 'NONE', ( #2157, #14322 ) ) ;
#24768=VERTEX_POINT ( 'NONE', #27821 ) ;
#24770=AXIS2_PLACEMENT_3D ( 'NONE', #26790, #14528, #3041 ) ;
#24820=DIRECTION ( 'NONE',  ( 1.000000000000000000, 0.000000000000000000, 0.000000000000000000 ) ) ;
#24837=VERTEX_POINT ( 'NONE', #4088 ) ;
#24877=ORIENTED_EDGE ( 'NONE', *, *, #13941, .T. ) ;
#24888=PRODUCT_DEFINITION_SHAPE ( 'NONE', 'NONE',  #24464 ) ;
#24958=B_SPLINE_CURVE_WITH_KNOTS ( 'NONE', 3,
 ( #2023, #21904, #16874, #2535 ),
 .UNSPECIFIED., .F., .F.,
 ( 4, 4 ),
 ( 0.9101643785142677912, 1.000000000000000000 ),
 .UNSPECIFIED. ) ;
#24973=DIRECTION ( 'NONE',  ( -1.000000000000000000, 0.000000000000000000, 0.000000000000000000 ) ) ;
#25006=ORIENTED_EDGE ( 'NONE', *, *, #19515, .F. ) ;
#25051=DIRECTION ( 'NONE',  ( 1.000000000000000000, 0.000000000000000000, 0.000000000000000000 ) ) ;
#25062=EDGE_CURVE ( 'NONE', #4592, #17515, #12845, .T. ) ;
#25078=CARTESIAN_POINT ( 'NONE',  ( -0.03937007874015747977, 0.000000000000000000, 0.000000000000000000 ) ) ;
#25097=DIRECTION ( 'NONE',  ( 1.000000000000000000, 0.000000000000000000, 0.000000000000000000 ) ) ;
#25117=CARTESIAN_POINT ( 'NONE',  ( -0.2362204724409449064, -0.4724409448818898127, -0.8182917201112815953 ) ) ;
#25133=ADVANCED_FACE ( 'NONE', ( #1644 ), #8014, .F. ) ;
#25135=LINE ( 'NONE', #25420, #6950 ) ;
#25144=LINE ( 'NONE', #20631, #2475 ) ;
#25162=COLOUR_RGB ( '', 0.31764706, 0.68627451, 0.89019608) ;
#25164=DIRECTION ( 'NONE',  ( 0.000000000000000000, 0.000000000000000000, 1.000000000000000000 ) ) ;
#25182=VERTEX_POINT ( 'NONE', #27784 ) ;
#25228=LINE ( 'NONE', #1777, #18533 ) ;
#25235=DIRECTION ( 'NONE',  ( 1.000000000000000000, 0.000000000000000000, 0.000000000000000000 ) ) ;
#25262=LINE ( 'NONE', #8448, #23342 ) ;
#25277=ADVANCED_FACE ( 'NONE', ( #25520, #21835 ), #8832, .T. ) ;
#25285=LINE ( 'NONE', #14858, #24306 ) ;
#25329=EDGE_CURVE ( 'NONE', #19874, #17373, #16137, .T. ) ;
#25358=CIRCLE ( 'NONE', #11380, 0.1308464566929133932 ) ;
#25407=AXIS2_PLACEMENT_3D ( 'NONE', #7024, #17348, #21998 ) ;
#25417=DIRECTION ( 'NONE',  ( 1.000000000000000000, 0.000000000000000000, 0.000000000000000000 ) ) ;
#25420=CARTESIAN_POINT ( 'NONE',  ( -0.03937007874015747977, -5.785732909357575061E-17, -0.4724409448818898127 ) ) ;
#25437=CARTESIAN_POINT ( 'NONE',  ( -0.02559055118110236185, 0.6299212598425196763, 0.000000000000000000 ) ) ;
#25442=ORIENTED_EDGE ( 'NONE', *, *, #928, .T. ) ;
#25467=VECTOR ( 'NONE', #21611, 39.37007874015748143 ) ;
#25489=FILL_AREA_STYLE ('',( #16881 ) ) ;
#25520=FACE_BOUND ( 'NONE', #25666, .T. ) ;
#25554=EDGE_LOOP ( 'NONE', ( #26039, #17739, #15001, #14419 ) ) ;
#25562=DIRECTION ( 'NONE',  ( 0.000000000000000000, 1.000000000000000000, 0.000000000000000000 ) ) ;
#25584=VERTEX_POINT ( 'NONE', #16407 ) ;
#25616=CARTESIAN_POINT ( 'NONE',  ( -0.6145047846951736670, -0.6192722590599607502, -0.9188490092316486946 ) ) ;
#25624=DIRECTION ( 'NONE',  ( 0.000000000000000000, 0.000000000000000000, -1.000000000000000000 ) ) ;
#25654=AXIS2_PLACEMENT_3D ( 'NONE', #22989, #20582, #18727 ) ;
#25666=EDGE_LOOP ( 'NONE', ( #10595, #2096 ) ) ;
#25678=AXIS2_PLACEMENT_3D ( 'NONE', #19814, #7102, #19950 ) ;
#25681=AXIS2_PLACEMENT_3D ( 'NONE', #12527, #25097, #16351 ) ;
#25709=ORIENTED_EDGE ( 'NONE', *, *, #2642, .F. ) ;
#25795=DIRECTION ( 'NONE',  ( -1.000000000000000000, 0.000000000000000000, 0.000000000000000000 ) ) ;
#25828=FACE_OUTER_BOUND ( 'NONE', #14801, .T. ) ;
#25830=ORIENTED_EDGE ( 'NONE', *, *, #24056, .T. ) ;
#25845=CARTESIAN_POINT ( 'NONE',  ( -0.03937007874015747977, 0.000000000000000000, 0.4724409448818898127 ) ) ;
#25853=CIRCLE ( 'NONE', #21342, 0.1308464566929133932 ) ;
#25856=ORIENTED_EDGE ( 'NONE', *, *, #24298, .F. ) ;
#25892=FACE_OUTER_BOUND ( 'NONE', #18776, .T. ) ;
#25909=EDGE_CURVE ( 'NONE', #3172, #9714, #11962, .T. ) ;
#25920=AXIS2_PLACEMENT_3D ( 'NONE', #20090, #9334, #26572 ) ;
#25951=EDGE_CURVE ( 'NONE', #25584, #25182, #6134, .T. ) ;
#25955=VERTEX_POINT ( 'NONE', #1989 ) ;
#26013=DIRECTION ( 'NONE',  ( 0.000000000000000000, 1.000000000000000000, 0.000000000000000000 ) ) ;
#26039=ORIENTED_EDGE ( 'NONE', *, *, #27146, .F. ) ;
#26049=CARTESIAN_POINT ( 'NONE',  ( -0.6299212598425196763, 0.000000000000000000, 0.000000000000000000 ) ) ;
#26050=CARTESIAN_POINT ( 'NONE',  ( -0.6212843287616266474, -0.6280845039693049303, 0.9045795100263914756 ) ) ;
#26053=AXIS2_PLACEMENT_3D ( 'NONE', #17180, #25795, #6443 ) ;
#26123=CARTESIAN_POINT ( 'NONE',  ( -0.05118110236220472370, 0.000000000000000000, 0.000000000000000000 ) ) ;
#26203=CARTESIAN_POINT ( 'NONE',  ( -0.01968503937007873988, 0.000000000000000000, 0.000000000000000000 ) ) ;
#26208=VECTOR ( 'NONE', #11219, 39.37007874015748143 ) ;
#26241=EDGE_LOOP ( 'NONE', ( #10282, #4033 ) ) ;
#26258=CYLINDRICAL_SURFACE ( 'NONE', #4929, 0.6299212598425196763 ) ;
#26286=DIRECTION ( 'NONE',  ( 1.000000000000000000, 0.000000000000000000, 0.000000000000000000 ) ) ;
#26305=CARTESIAN_POINT ( 'NONE',  ( 2.632951206231566310, 0.9448818897637796255, 0.1308464566929133654 ) ) ;
#26308=CARTESIAN_POINT ( 'NONE',  ( -0.1141732283464566844, 0.000000000000000000, 0.000000000000000000 ) ) ;
#26323=LINE ( 'NONE', #11080, #18695 ) ;
#26324=PLANE ( 'NONE',  #16501 ) ;
#26342=ORIENTED_EDGE ( 'NONE', *, *, #6294, .F. ) ;
#26361=ORIENTED_EDGE ( 'NONE', *, *, #12383, .T. ) ;
#26427=ORIENTED_EDGE ( 'NONE', *, *, #15192, .F. ) ;
#26443=AXIS2_PLACEMENT_3D ( 'NONE', #18581, #2609, #20041 ) ;
#26462=DIRECTION ( 'NONE',  ( 0.000000000000000000, 0.000000000000000000, 1.000000000000000000 ) ) ;
#26477=AXIS2_PLACEMENT_3D ( 'NONE', #24222, #16028, #2600 ) ;
#26491=CARTESIAN_POINT ( 'NONE',  ( -0.6102362204724409711, 0.000000000000000000, 0.000000000000000000 ) ) ;
#26494=VERTEX_POINT ( 'NONE', #13708 ) ;
#26523=ORIENTED_EDGE ( 'NONE', *, *, #15727, .F. ) ;
#26533=AXIS2_PLACEMENT_3D ( 'NONE', #4499, #4227, #21463 ) ;
#26561=VERTEX_POINT ( 'NONE', #9053 ) ;
#26572=DIRECTION ( 'NONE',  ( 0.000000000000000000, 0.000000000000000000, 1.000000000000000000 ) ) ;
#26587=CARTESIAN_POINT ( 'NONE',  ( -0.5177165354330708347, 0.9448818897637796255, -9.561468503937007847E-18 ) ) ;
#26604=CARTESIAN_POINT ( 'NONE',  ( -0.2362204724409449064, 0.000000000000000000, 0.000000000000000000 ) ) ;
#26638=ORIENTED_EDGE ( 'NONE', *, *, #6004, .F. ) ;
#26641=CYLINDRICAL_SURFACE ( 'NONE', #4100, 0.1771653543307086798 ) ;
#26657=AXIS2_PLACEMENT_3D ( 'NONE', #7541, #1198, #26462 ) ;
#26685=CARTESIAN_POINT ( 'NONE',  ( -0.05118110236220472370, 0.000000000000000000, 0.000000000000000000 ) ) ;
#26741=DIRECTION ( 'NONE',  ( 1.000000000000000000, 0.000000000000000000, 0.000000000000000000 ) ) ;
#26757=ORIENTED_EDGE ( 'NONE', *, *, #5617, .F. ) ;
#26770=AXIS2_PLACEMENT_3D ( 'NONE', #12565, #25417, #25562 ) ;
#26778=CARTESIAN_POINT ( 'NONE',  ( -0.4055118110236220486, 0.9448818897637796255, -0.1308464566929134210 ) ) ;
#26790=CARTESIAN_POINT ( 'NONE',  ( -0.1771653543307086520, 0.000000000000000000, 0.000000000000000000 ) ) ;
#26832=UNCERTAINTY_MEASURE_WITH_UNIT (LENGTH_MEASURE( 1.000000000000000082E-05 ), #24681, 'distance_accuracy_value', 'NONE') ;
#26863=CIRCLE ( 'NONE', #7470, 1.092519685039370136 ) ;
#26868=VERTEX_POINT ( 'NONE', #21053 ) ;
#26888=FACE_OUTER_BOUND ( 'NONE', #22008, .T. ) ;
#26925=DIRECTION ( 'NONE',  ( 1.000000000000000000, 0.000000000000000000, 0.000000000000000000 ) ) ;
#26930=DIRECTION ( 'NONE',  ( 0.000000000000000000, 0.000000000000000000, 1.000000000000000000 ) ) ;
#26973=DIRECTION ( 'NONE',  ( -1.000000000000000000, 0.000000000000000000, 0.000000000000000000 ) ) ;
#27003=EDGE_LOOP ( 'NONE', ( #14735, #18843 ) ) ;
#27083=CYLINDRICAL_SURFACE ( 'NONE', #25654, 1.131889763779527547 ) ;
#27088=AXIS2_PLACEMENT_3D ( 'NONE', #22170, #26973, #7623 ) ;
#27108=FACE_BOUND ( 'NONE', #19305, .T. ) ;
#27139=CARTESIAN_POINT ( 'NONE',  ( 1.857656692913385893E-16, 0.000000000000000000, 0.000000000000000000 ) ) ;
#27146=EDGE_CURVE ( 'NONE', #13695, #27811, #25262, .T. ) ;
#27163=DIRECTION ( 'NONE',  ( 0.000000000000000000, 0.000000000000000000, -1.000000000000000000 ) ) ;
#27212=ORIENTED_EDGE ( 'NONE', *, *, #2720, .T. ) ;
#27250=VERTEX_POINT ( 'NONE', #2630 ) ;
#27350=ORIENTED_EDGE ( 'NONE', *, *, #10208, .F. ) ;
#27438=EDGE_CURVE ( 'NONE', #10695, #12956, #9796, .T. ) ;
#27440=CARTESIAN_POINT ( 'NONE',  ( -0.2362204724409449064, 0.9448818897637796255, -9.561468503937007847E-18 ) ) ;
#27441=ORIENTED_EDGE ( 'NONE', *, *, #12347, .T. ) ;
#27457=CARTESIAN_POINT ( 'NONE',  ( -0.6054097002486862333, -0.5184600247616719670, -0.9894322414030318757 ) ) ;
#27458=VECTOR ( 'NONE', #1701, 39.37007874015748143 ) ;
#27466=CARTESIAN_POINT ( 'NONE',  ( -0.6102362204724409711, 0.000000000000000000, 0.000000000000000000 ) ) ;
#27475=ADVANCED_FACE ( 'NONE', ( #913 ), #11630, .F. ) ;
#27483=ADVANCED_FACE ( 'NONE', ( #26888 ), #16166, .T. ) ;
#27520=AXIS2_PLACEMENT_3D ( 'NONE', #26203, #10959, #17974 ) ;
#27556=CARTESIAN_POINT ( 'NONE',  ( -0.1771653543307086520, 0.000000000000000000, 0.000000000000000000 ) ) ;
#27564=AXIS2_PLACEMENT_3D ( 'NONE', #3458, #18284, #26930 ) ;
#27569=CARTESIAN_POINT ( 'NONE',  ( -0.5177165354330708347, -0.4724409448818898127, -0.6411263657805729155 ) ) ;
#27615=CIRCLE ( 'NONE', #22188, 1.092519685039370136 ) ;
#27634=EDGE_LOOP ( 'NONE', ( #4704, #3017, #9178, #1346 ) ) ;
#27661=ORIENTED_EDGE ( 'NONE', *, *, #24629, .F. ) ;
#27691=AXIS2_PLACEMENT_3D ( 'NONE', #25078, #26925, #3169 ) ;
#27709=ADVANCED_FACE ( 'NONE', ( #10882 ), #19497, .F. ) ;
#27746=CARTESIAN_POINT ( 'NONE',  ( -0.6212848329275697523, -0.6280848967520035186, -0.9045786101299029269 ) ) ;
#27753=DIRECTION ( 'NONE',  ( 0.000000000000000000, -1.000000000000000000, 0.000000000000000000 ) ) ;
#27768=CARTESIAN_POINT ( 'NONE',  ( -0.6003337592290733937, -0.5548708868587087784, 0.9753553170054337640 ) ) ;
#27784=CARTESIAN_POINT ( 'NONE',  ( -0.03937007874015747977, 0.6299212598425196763, 0.000000000000000000 ) ) ;
#27800=ADVANCED_FACE ( 'NONE', ( #6196 ), #2955, .T. ) ;
#27811=VERTEX_POINT ( 'NONE', #3919 ) ;
#27817=ORIENTED_EDGE ( 'NONE', *, *, #6805, .T. ) ;
#27821=CARTESIAN_POINT ( 'NONE',  ( -0.4055118110236220486, -0.4724409448818898127, 0.6411263657805708061 ) ) ;
#27861=DIRECTION ( 'NONE',  ( 1.000000000000000000, 0.000000000000000000, 0.000000000000000000 ) ) ;
#27868=CARTESIAN_POINT ( 'NONE',  ( -0.5177165354330708347, -0.4724409448818898127, -0.9954570744419902750 ) ) ;
ENDSEC;
END-ISO-10303-21;
